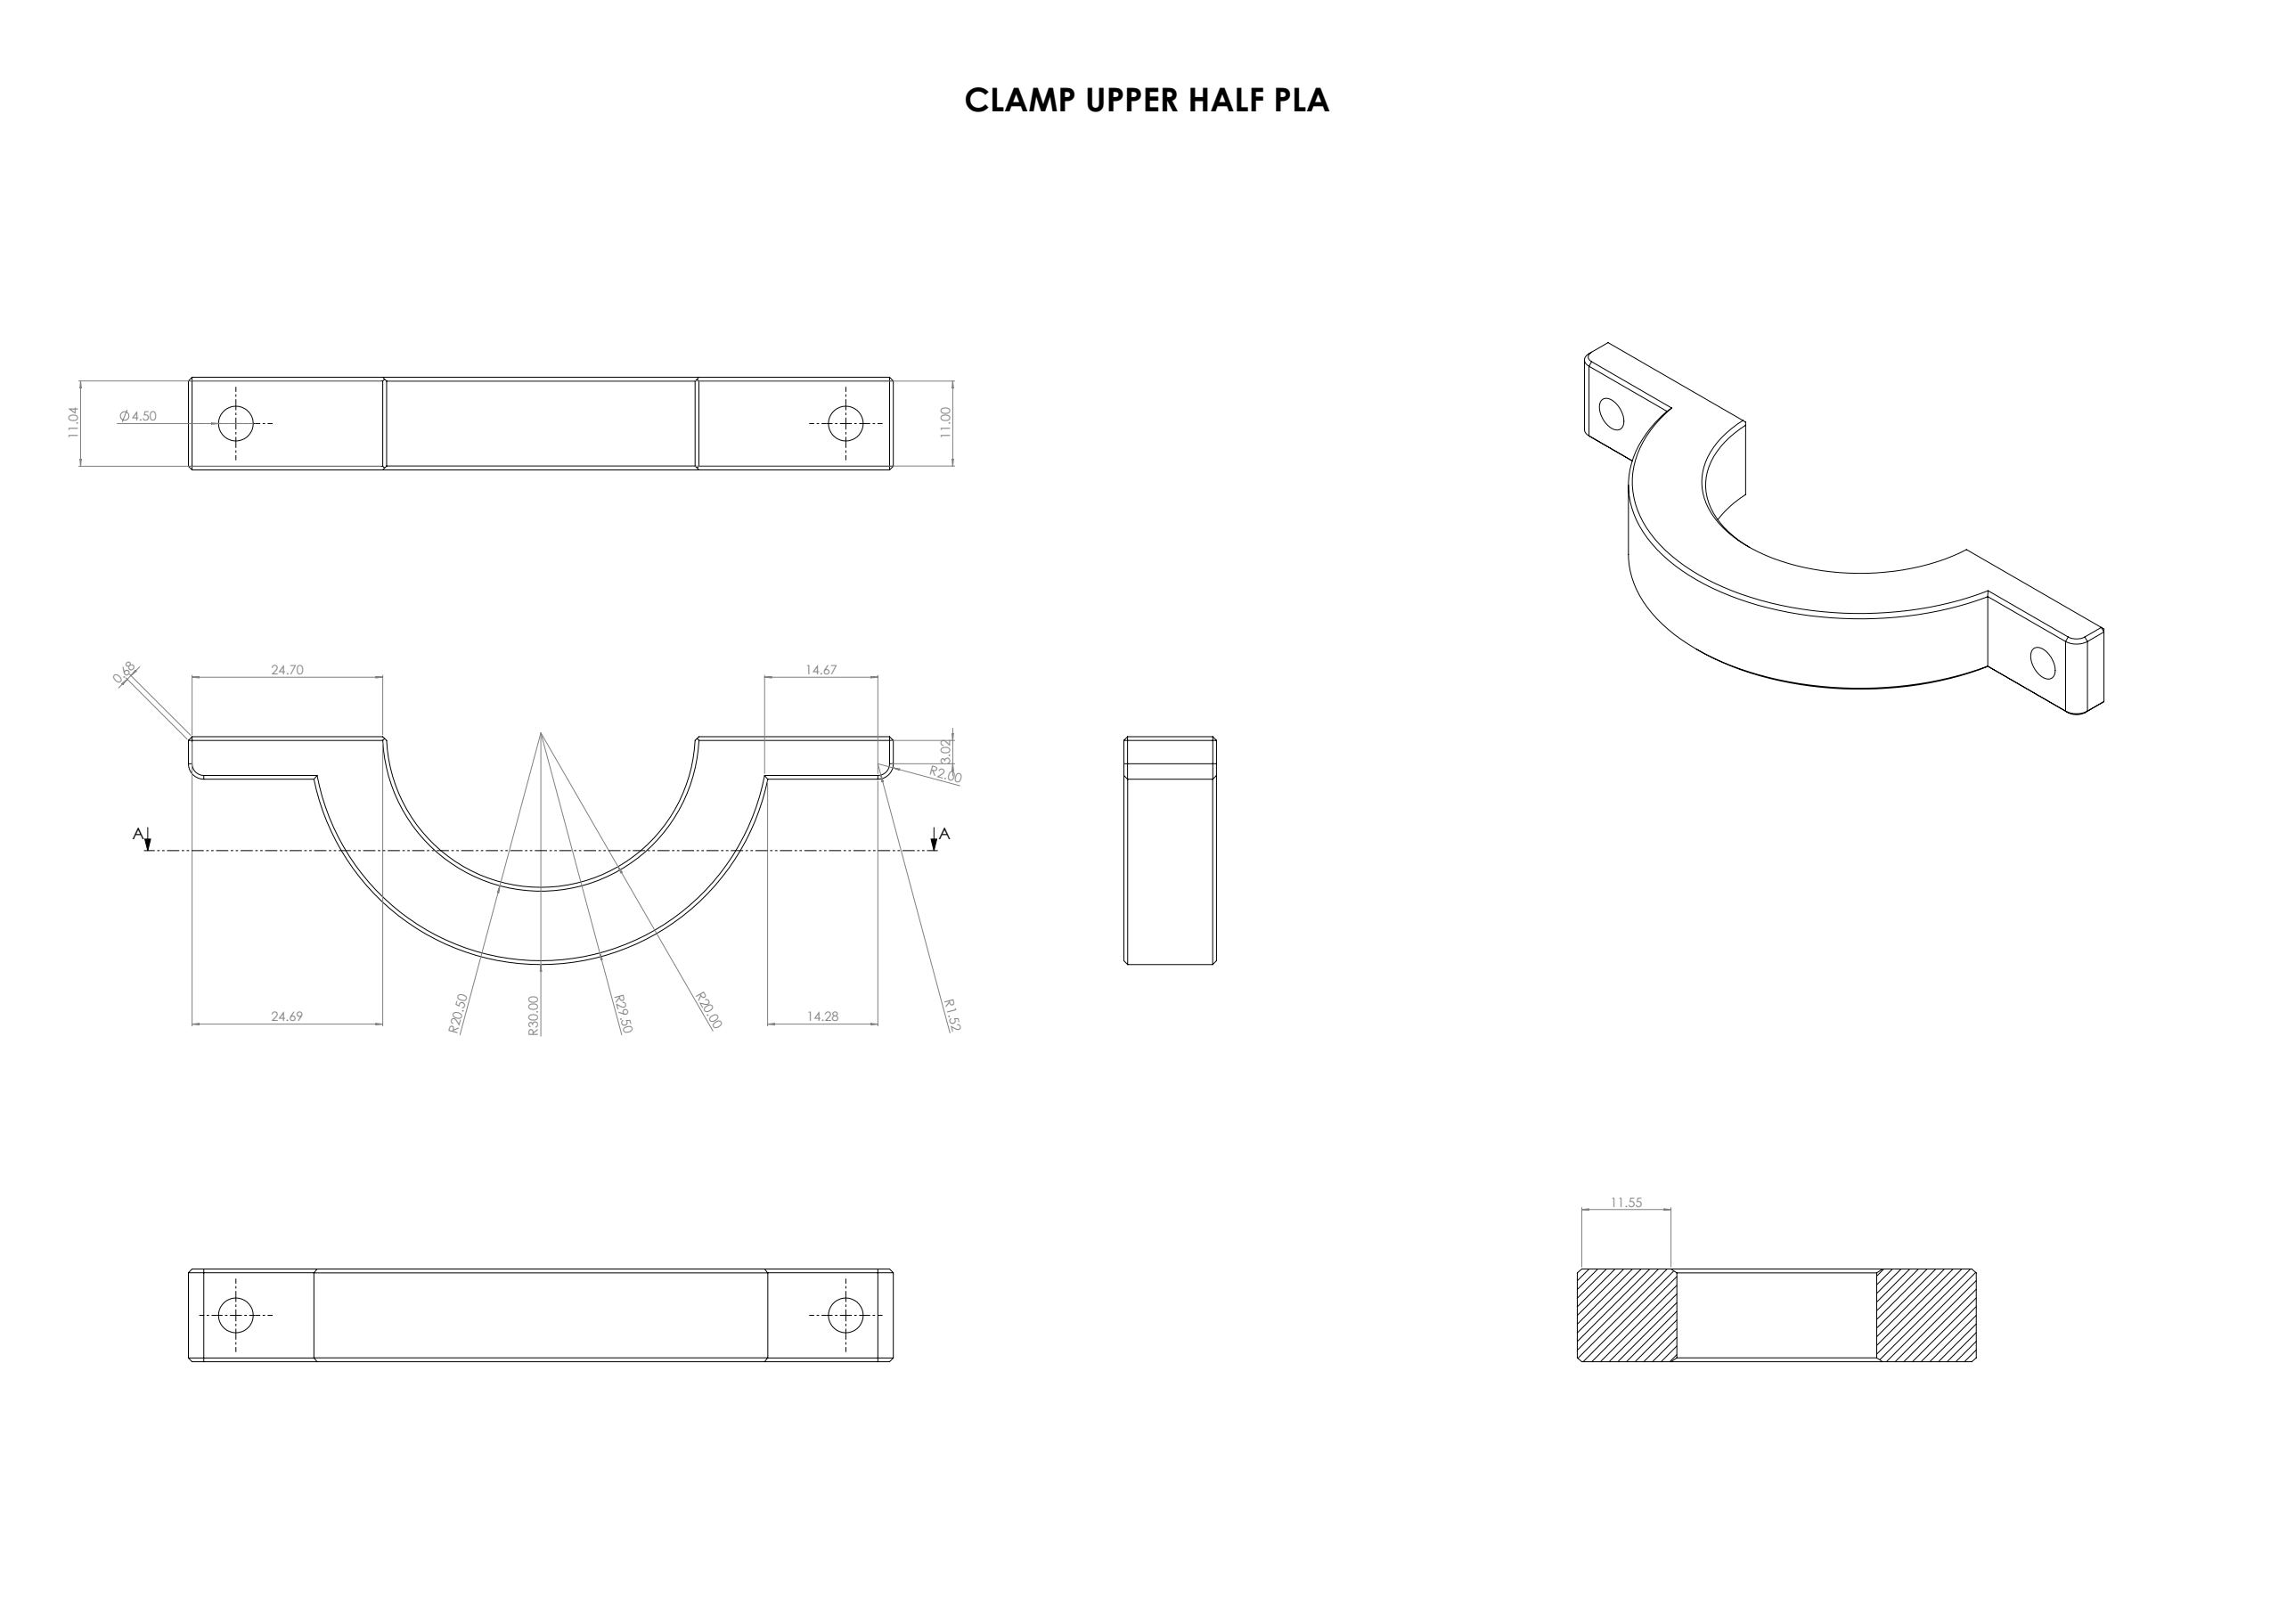
ISO-10303-21;
HEADER;
/* Generated by software containing ST-Developer
 * from STEP Tools, Inc. (www.steptools.com) 
 */

FILE_DESCRIPTION(
/* description */ (''),
/* implementation_level */ '2;1');

FILE_NAME(
/* name */ '01_Clamp_Upper_Half_PLA.step',
/* time_stamp */ '2026-10-21T02:01:14-07:00',
/* author */ (''),
/* organization */ (''),
/* preprocessor_version */ 'ST-DEVELOPER v20.2',
/* originating_system */ 'Autodesk Translation Framework v15.15.0.0',
/* authorisation */ '');

FILE_SCHEMA (('AUTOMOTIVE_DESIGN { 1 0 10303 214 3 1 1 }'));
ENDSEC;

DATA;
#10=MECHANICAL_DESIGN_GEOMETRIC_PRESENTATION_REPRESENTATION('',(#614),#37181);
#588=SHAPE_REPRESENTATION_RELATIONSHIP('SRR','None',#37238,#601);
#601=ADVANCED_BREP_SHAPE_REPRESENTATION('',(#627),#37168);
#614=STYLED_ITEM('',(#37359),#627);
#627=MANIFOLD_SOLID_BREP('Body1',#14776);
#640=FACE_BOUND('',#2226,.T.);
#641=FACE_BOUND('',#2241,.T.);
#642=FACE_BOUND('',#2250,.T.);
#643=FACE_BOUND('',#2253,.T.);
#690=CYLINDRICAL_SURFACE('',#14940,20.);
#691=CYLINDRICAL_SURFACE('',#14961,2.);
#692=CYLINDRICAL_SURFACE('',#14987,30.);
#693=CYLINDRICAL_SURFACE('',#14988,2.25);
#694=CYLINDRICAL_SURFACE('',#14990,2.25);
#695=CYLINDRICAL_SURFACE('',#14993,2.);
#951=CIRCLE('',#14938,20.);
#952=CIRCLE('',#14939,20.5);
#953=CIRCLE('',#14941,20.);
#954=CIRCLE('',#14946,2.);
#955=CIRCLE('',#14947,1.52);
#956=CIRCLE('',#14953,2.);
#957=CIRCLE('',#14954,1.52);
#958=CIRCLE('',#14957,29.5);
#959=CIRCLE('',#14958,1.52);
#960=CIRCLE('',#14959,20.5);
#961=CIRCLE('',#14963,2.25);
#962=CIRCLE('',#14971,2.);
#963=CIRCLE('',#14976,2.);
#964=CIRCLE('',#14977,1.52);
#965=CIRCLE('',#14981,2.25);
#966=CIRCLE('',#14983,30.);
#967=CIRCLE('',#14985,30.);
#968=CIRCLE('',#14986,29.5);
#969=CIRCLE('',#14989,2.25);
#970=CIRCLE('',#14991,2.25);
#1283=CONICAL_SURFACE('',#14937,20.25,0.785398163397446);
#1284=CONICAL_SURFACE('',#14945,1.76,0.78539816339745);
#1285=CONICAL_SURFACE('',#14952,1.76,0.78539816339745);
#1286=CONICAL_SURFACE('',#14970,1.76,0.785398163397452);
#1287=CONICAL_SURFACE('',#14975,1.76,0.785398163397452);
#1288=CONICAL_SURFACE('',#14979,20.25,0.785398163397446);
#1289=CONICAL_SURFACE('',#14982,29.75,0.785398163397446);
#1290=CONICAL_SURFACE('',#14984,29.75,0.785398163397446);
#1368=FACE_OUTER_BOUND('',#2208,.T.);
#1369=FACE_OUTER_BOUND('',#2209,.T.);
#1370=FACE_OUTER_BOUND('',#2210,.T.);
#1371=FACE_OUTER_BOUND('',#2211,.T.);
#1372=FACE_OUTER_BOUND('',#2212,.T.);
#1373=FACE_OUTER_BOUND('',#2213,.T.);
#1374=FACE_OUTER_BOUND('',#2214,.T.);
#1375=FACE_OUTER_BOUND('',#2215,.T.);
#1376=FACE_OUTER_BOUND('',#2216,.T.);
#1377=FACE_OUTER_BOUND('',#2217,.T.);
#1378=FACE_OUTER_BOUND('',#2218,.T.);
#1379=FACE_OUTER_BOUND('',#2219,.T.);
#1380=FACE_OUTER_BOUND('',#2220,.T.);
#1381=FACE_OUTER_BOUND('',#2221,.T.);
#1382=FACE_OUTER_BOUND('',#2222,.T.);
#1383=FACE_OUTER_BOUND('',#2223,.T.);
#1384=FACE_OUTER_BOUND('',#2224,.T.);
#1385=FACE_OUTER_BOUND('',#2225,.T.);
#1386=FACE_OUTER_BOUND('',#2227,.T.);
#1387=FACE_OUTER_BOUND('',#2228,.T.);
#1388=FACE_OUTER_BOUND('',#2229,.T.);
#1389=FACE_OUTER_BOUND('',#2230,.T.);
#1390=FACE_OUTER_BOUND('',#2231,.T.);
#1391=FACE_OUTER_BOUND('',#2232,.T.);
#1392=FACE_OUTER_BOUND('',#2233,.T.);
#1393=FACE_OUTER_BOUND('',#2234,.T.);
#1394=FACE_OUTER_BOUND('',#2235,.T.);
#1395=FACE_OUTER_BOUND('',#2236,.T.);
#1396=FACE_OUTER_BOUND('',#2237,.T.);
#1397=FACE_OUTER_BOUND('',#2238,.T.);
#1398=FACE_OUTER_BOUND('',#2239,.T.);
#1399=FACE_OUTER_BOUND('',#2240,.T.);
#1400=FACE_OUTER_BOUND('',#2242,.T.);
#1401=FACE_OUTER_BOUND('',#2243,.T.);
#1402=FACE_OUTER_BOUND('',#2244,.T.);
#1403=FACE_OUTER_BOUND('',#2245,.T.);
#1404=FACE_OUTER_BOUND('',#2246,.T.);
#1405=FACE_OUTER_BOUND('',#2247,.T.);
#1406=FACE_OUTER_BOUND('',#2248,.T.);
#1407=FACE_OUTER_BOUND('',#2249,.T.);
#1408=FACE_OUTER_BOUND('',#2251,.T.);
#1409=FACE_OUTER_BOUND('',#2252,.T.);
#2208=EDGE_LOOP('',(#9171,#9172,#9173,#9174,#9175,#9176));
#2209=EDGE_LOOP('',(#9177,#9178,#9179,#9180,#9181));
#2210=EDGE_LOOP('',(#9182,#9183,#9184,#9185,#9186,#9187));
#2211=EDGE_LOOP('',(#9188,#9189,#9190,#9191));
#2212=EDGE_LOOP('',(#9192,#9193,#9194));
#2213=EDGE_LOOP('',(#9195,#9196,#9197));
#2214=EDGE_LOOP('',(#9198,#9199,#9200,#9201));
#2215=EDGE_LOOP('',(#9202,#9203,#9204,#9205));
#2216=EDGE_LOOP('',(#9206,#9207,#9208,#9209));
#2217=EDGE_LOOP('',(#9210,#9211,#9212,#9213,#9214));
#2218=EDGE_LOOP('',(#9215,#9216,#9217,#9218));
#2219=EDGE_LOOP('',(#9219,#9220,#9221,#9222));
#2220=EDGE_LOOP('',(#9223,#9224,#9225,#9226));
#2221=EDGE_LOOP('',(#9227,#9228,#9229,#9230));
#2222=EDGE_LOOP('',(#9231,#9232,#9233,#9234,#9235,#9236,#9237,#9238,#9239,
#9240));
#2223=EDGE_LOOP('',(#9241,#9242,#9243,#9244));
#2224=EDGE_LOOP('',(#9245,#9246,#9247,#9248));
#2225=EDGE_LOOP('',(#9249,#9250,#9251,#9252,#9253,#9254));
#2226=EDGE_LOOP('',(#9255));
#2227=EDGE_LOOP('',(#9256,#9257,#9258,#9259,#9260,#9261));
#2228=EDGE_LOOP('',(#9262,#9263,#9264,#9265,#9266));
#2229=EDGE_LOOP('',(#9267,#9268,#9269));
#2230=EDGE_LOOP('',(#9270,#9271,#9272));
#2231=EDGE_LOOP('',(#9273,#9274,#9275,#9276,#9277));
#2232=EDGE_LOOP('',(#9278,#9279,#9280,#9281));
#2233=EDGE_LOOP('',(#9282,#9283,#9284,#9285));
#2234=EDGE_LOOP('',(#9286,#9287,#9288,#9289));
#2235=EDGE_LOOP('',(#9290,#9291,#9292,#9293));
#2236=EDGE_LOOP('',(#9294,#9295,#9296,#9297));
#2237=EDGE_LOOP('',(#9298,#9299,#9300,#9301));
#2238=EDGE_LOOP('',(#9302,#9303,#9304,#9305));
#2239=EDGE_LOOP('',(#9306,#9307,#9308,#9309,#9310,#9311));
#2240=EDGE_LOOP('',(#9312,#9313,#9314,#9315));
#2241=EDGE_LOOP('',(#9316));
#2242=EDGE_LOOP('',(#9317,#9318,#9319,#9320,#9321,#9322));
#2243=EDGE_LOOP('',(#9323,#9324,#9325,#9326,#9327,#9328));
#2244=EDGE_LOOP('',(#9329,#9330,#9331,#9332));
#2245=EDGE_LOOP('',(#9333,#9334,#9335,#9336));
#2246=EDGE_LOOP('',(#9337,#9338,#9339,#9340));
#2247=EDGE_LOOP('',(#9341,#9342,#9343,#9344,#9345,#9346,#9347,#9348,#9349,
#9350));
#2248=EDGE_LOOP('',(#9351,#9352,#9353,#9354));
#2249=EDGE_LOOP('',(#9355,#9356,#9357,#9358,#9359,#9360));
#2250=EDGE_LOOP('',(#9361));
#2251=EDGE_LOOP('',(#9362,#9363,#9364,#9365));
#2252=EDGE_LOOP('',(#9366,#9367,#9368,#9369));
#2253=EDGE_LOOP('',(#9370));
#3098=(
BOUNDED_CURVE()
B_SPLINE_CURVE(2,(#19759,#19760,#19761),.UNSPECIFIED.,.F.,.F.)
B_SPLINE_CURVE_WITH_KNOTS((3,3),(0.0434191036447886,0.0876516150043351),
 .UNSPECIFIED.)
CURVE()
GEOMETRIC_REPRESENTATION_ITEM()
RATIONAL_B_SPLINE_CURVE((1.00007900493244,1.00007974496639,1.))
REPRESENTATION_ITEM('')
);
#3099=(
BOUNDED_CURVE()
B_SPLINE_CURVE(2,(#19764,#19765,#19766),.UNSPECIFIED.,.F.,.F.)
B_SPLINE_CURVE_WITH_KNOTS((3,3),(0.,0.0442325113595662),.UNSPECIFIED.)
CURVE()
GEOMETRIC_REPRESENTATION_ITEM()
RATIONAL_B_SPLINE_CURVE((1.,1.00007974496581,1.00007900493187))
REPRESENTATION_ITEM('')
);
#3100=(
BOUNDED_CURVE()
B_SPLINE_CURVE(2,(#19769,#19770,#19771),.UNSPECIFIED.,.F.,.F.)
B_SPLINE_CURVE_WITH_KNOTS((3,3),(0.0429017134859095,0.085594459730905),
 .UNSPECIFIED.)
CURVE()
GEOMETRIC_REPRESENTATION_ITEM()
RATIONAL_B_SPLINE_CURVE((1.,1.,1.))
REPRESENTATION_ITEM('')
);
#3101=(
BOUNDED_CURVE()
B_SPLINE_CURVE(2,(#19781,#19782,#19783),.UNSPECIFIED.,.F.,.F.)
B_SPLINE_CURVE_WITH_KNOTS((3,3),(0.0434191036447867,0.0876516150043353),
 .UNSPECIFIED.)
CURVE()
GEOMETRIC_REPRESENTATION_ITEM()
RATIONAL_B_SPLINE_CURVE((1.00007900493282,1.00007974496678,1.))
REPRESENTATION_ITEM('')
);
#3102=(
BOUNDED_CURVE()
B_SPLINE_CURVE(2,(#19785,#19786,#19787),.UNSPECIFIED.,.F.,.F.)
B_SPLINE_CURVE_WITH_KNOTS((3,3),(0.,0.0426927462450535),.UNSPECIFIED.)
CURVE()
GEOMETRIC_REPRESENTATION_ITEM()
RATIONAL_B_SPLINE_CURVE((1.,1.,1.))
REPRESENTATION_ITEM('')
);
#3103=(
BOUNDED_CURVE()
B_SPLINE_CURVE(2,(#19819,#19820,#19821),.UNSPECIFIED.,.F.,.F.)
B_SPLINE_CURVE_WITH_KNOTS((3,3),(0.,0.0785138217700896),.UNSPECIFIED.)
CURVE()
GEOMETRIC_REPRESENTATION_ITEM()
RATIONAL_B_SPLINE_CURVE((1.,1.,1.))
REPRESENTATION_ITEM('')
);
#3104=(
BOUNDED_CURVE()
B_SPLINE_CURVE(2,(#19828,#19829,#19830),.UNSPECIFIED.,.F.,.F.)
B_SPLINE_CURVE_WITH_KNOTS((3,3),(0.,0.0426927462450536),.UNSPECIFIED.)
CURVE()
GEOMETRIC_REPRESENTATION_ITEM()
RATIONAL_B_SPLINE_CURVE((1.,1.,1.))
REPRESENTATION_ITEM('')
);
#3105=(
BOUNDED_CURVE()
B_SPLINE_CURVE(2,(#19837,#19838,#19839),.UNSPECIFIED.,.F.,.F.)
B_SPLINE_CURVE_WITH_KNOTS((3,3),(0.,0.0785138217700896),.UNSPECIFIED.)
CURVE()
GEOMETRIC_REPRESENTATION_ITEM()
RATIONAL_B_SPLINE_CURVE((1.,1.,1.))
REPRESENTATION_ITEM('')
);
#3106=(
BOUNDED_CURVE()
B_SPLINE_CURVE(2,(#19872,#19873,#19874),.UNSPECIFIED.,.F.,.F.)
B_SPLINE_CURVE_WITH_KNOTS((3,3),(0.0686220150831262,0.071456332389423),
 .UNSPECIFIED.)
CURVE()
GEOMETRIC_REPRESENTATION_ITEM()
RATIONAL_B_SPLINE_CURVE((1.00000280409598,1.00000145995723,1.))
REPRESENTATION_ITEM('')
);
#3107=(
BOUNDED_CURVE()
B_SPLINE_CURVE(2,(#19877,#19878,#19879),.UNSPECIFIED.,.F.,.F.)
B_SPLINE_CURVE_WITH_KNOTS((3,3),(0.,0.00283431730629652),.UNSPECIFIED.)
CURVE()
GEOMETRIC_REPRESENTATION_ITEM()
RATIONAL_B_SPLINE_CURVE((1.,1.00000145995723,1.00000280409598))
REPRESENTATION_ITEM('')
);
#3108=(
BOUNDED_CURVE()
B_SPLINE_CURVE(2,(#19889,#19890,#19891),.UNSPECIFIED.,.F.,.F.)
B_SPLINE_CURVE_WITH_KNOTS((3,3),(0.,0.0442325113595461),.UNSPECIFIED.)
CURVE()
GEOMETRIC_REPRESENTATION_ITEM()
RATIONAL_B_SPLINE_CURVE((1.,1.00007974496639,1.00007900493244))
REPRESENTATION_ITEM('')
);
#3109=(
BOUNDED_CURVE()
B_SPLINE_CURVE(2,(#19909,#19910,#19911),.UNSPECIFIED.,.F.,.F.)
B_SPLINE_CURVE_WITH_KNOTS((3,3),(0.0429017134859048,0.0855944597309048),
 .UNSPECIFIED.)
CURVE()
GEOMETRIC_REPRESENTATION_ITEM()
RATIONAL_B_SPLINE_CURVE((1.,1.,1.))
REPRESENTATION_ITEM('')
);
#3110=(
BOUNDED_CURVE()
B_SPLINE_CURVE(2,(#19915,#19916,#19917),.UNSPECIFIED.,.F.,.F.)
B_SPLINE_CURVE_WITH_KNOTS((3,3),(0.,0.0785138217700896),.UNSPECIFIED.)
CURVE()
GEOMETRIC_REPRESENTATION_ITEM()
RATIONAL_B_SPLINE_CURVE((1.,1.,1.))
REPRESENTATION_ITEM('')
);
#3111=(
BOUNDED_CURVE()
B_SPLINE_CURVE(2,(#19945,#19946,#19947),.UNSPECIFIED.,.F.,.F.)
B_SPLINE_CURVE_WITH_KNOTS((3,3),(0.,0.0785138217700896),.UNSPECIFIED.)
CURVE()
GEOMETRIC_REPRESENTATION_ITEM()
RATIONAL_B_SPLINE_CURVE((1.,1.,1.))
REPRESENTATION_ITEM('')
);
#3112=(
BOUNDED_CURVE()
B_SPLINE_CURVE(2,(#19956,#19957,#19958),.UNSPECIFIED.,.F.,.F.)
B_SPLINE_CURVE_WITH_KNOTS((3,3),(0.0686220150831262,0.071456332389423),
 .UNSPECIFIED.)
CURVE()
GEOMETRIC_REPRESENTATION_ITEM()
RATIONAL_B_SPLINE_CURVE((1.00000280409598,1.00000145995723,1.))
REPRESENTATION_ITEM('')
);
#3113=(
BOUNDED_CURVE()
B_SPLINE_CURVE(2,(#19962,#19963,#19964),.UNSPECIFIED.,.F.,.F.)
B_SPLINE_CURVE_WITH_KNOTS((3,3),(0.,0.00283431730629652),.UNSPECIFIED.)
CURVE()
GEOMETRIC_REPRESENTATION_ITEM()
RATIONAL_B_SPLINE_CURVE((1.,1.00000145995723,1.00000280409598))
REPRESENTATION_ITEM('')
);
#3203=LINE('',#19753,#4442);
#3204=LINE('',#19755,#4443);
#3205=LINE('',#19757,#4444);
#3206=LINE('',#19763,#4445);
#3207=LINE('',#19773,#4446);
#3208=LINE('',#19775,#4447);
#3209=LINE('',#19776,#4448);
#3210=LINE('',#19792,#4449);
#3211=LINE('',#19795,#4450);
#3212=LINE('',#19796,#4451);
#3213=LINE('',#19800,#4452);
#3214=LINE('',#19802,#4453);
#3215=LINE('',#19803,#4454);
#3216=LINE('',#19807,#4455);
#3217=LINE('',#19808,#4456);
#3218=LINE('',#19809,#4457);
#3219=LINE('',#19814,#4458);
#3220=LINE('',#19822,#4459);
#3221=LINE('',#19823,#4460);
#3222=LINE('',#19825,#4461);
#3223=LINE('',#19827,#4462);
#3224=LINE('',#19832,#4463);
#3225=LINE('',#19833,#4464);
#3226=LINE('',#19841,#4465);
#3227=LINE('',#19843,#4466);
#3228=LINE('',#19844,#4467);
#3229=LINE('',#19849,#4468);
#3230=LINE('',#19852,#4469);
#3231=LINE('',#19853,#4470);
#3232=LINE('',#19858,#4471);
#3233=LINE('',#19862,#4472);
#3234=LINE('',#19864,#4473);
#3235=LINE('',#19867,#4474);
#3236=LINE('',#19869,#4475);
#3237=LINE('',#19876,#4476);
#3238=LINE('',#19885,#4477);
#3239=LINE('',#19887,#4478);
#3240=LINE('',#19888,#4479);
#3241=LINE('',#19894,#4480);
#3242=LINE('',#19896,#4481);
#3243=LINE('',#19897,#4482);
#3244=LINE('',#19900,#4483);
#3245=LINE('',#19901,#4484);
#3246=LINE('',#19905,#4485);
#3247=LINE('',#19906,#4486);
#3248=LINE('',#19907,#4487);
#3249=LINE('',#19912,#4488);
#3250=LINE('',#19919,#4489);
#3251=LINE('',#19920,#4490);
#3252=LINE('',#19924,#4491);
#3253=LINE('',#19926,#4492);
#3254=LINE('',#19928,#4493);
#3255=LINE('',#19929,#4494);
#3256=LINE('',#19933,#4495);
#3257=LINE('',#19934,#4496);
#3258=LINE('',#19935,#4497);
#3259=LINE('',#19940,#4498);
#3260=LINE('',#19948,#4499);
#3261=LINE('',#19949,#4500);
#3262=LINE('',#19968,#4501);
#3263=LINE('',#19971,#4502);
#3264=LINE('',#19976,#4503);
#3265=LINE('',#19979,#4504);
#3266=LINE('',#19980,#4505);
#4442=VECTOR('',#16131,10.);
#4443=VECTOR('',#16132,10.);
#4444=VECTOR('',#16133,10.);
#4445=VECTOR('',#16134,10.);
#4446=VECTOR('',#16137,10.);
#4447=VECTOR('',#16138,10.);
#4448=VECTOR('',#16139,10.);
#4449=VECTOR('',#16150,10.);
#4450=VECTOR('',#16153,10.);
#4451=VECTOR('',#16154,10.);
#4452=VECTOR('',#16157,10.);
#4453=VECTOR('',#16158,10.);
#4454=VECTOR('',#16159,10.);
#4455=VECTOR('',#16162,10.);
#4456=VECTOR('',#16163,10.);
#4457=VECTOR('',#16164,10.);
#4458=VECTOR('',#16169,10.);
#4459=VECTOR('',#16174,10.);
#4460=VECTOR('',#16175,10.);
#4461=VECTOR('',#16178,10.);
#4462=VECTOR('',#16179,10.);
#4463=VECTOR('',#16182,10.);
#4464=VECTOR('',#16183,10.);
#4465=VECTOR('',#16186,10.);
#4466=VECTOR('',#16187,10.);
#4467=VECTOR('',#16188,10.);
#4468=VECTOR('',#16193,10.);
#4469=VECTOR('',#16198,10.);
#4470=VECTOR('',#16199,10.);
#4471=VECTOR('',#16204,10.);
#4472=VECTOR('',#16207,10.);
#4473=VECTOR('',#16208,10.);
#4474=VECTOR('',#16213,10.);
#4475=VECTOR('',#16216,10.);
#4476=VECTOR('',#16219,10.);
#4477=VECTOR('',#16224,10.);
#4478=VECTOR('',#16225,10.);
#4479=VECTOR('',#16226,10.);
#4480=VECTOR('',#16229,10.);
#4481=VECTOR('',#16230,10.);
#4482=VECTOR('',#16231,10.);
#4483=VECTOR('',#16234,10.);
#4484=VECTOR('',#16235,10.);
#4485=VECTOR('',#16238,10.);
#4486=VECTOR('',#16239,10.);
#4487=VECTOR('',#16240,10.);
#4488=VECTOR('',#16243,10.);
#4489=VECTOR('',#16246,10.);
#4490=VECTOR('',#16247,10.);
#4491=VECTOR('',#16252,10.);
#4492=VECTOR('',#16255,10.);
#4493=VECTOR('',#16258,10.);
#4494=VECTOR('',#16259,10.);
#4495=VECTOR('',#16262,10.);
#4496=VECTOR('',#16263,10.);
#4497=VECTOR('',#16264,10.);
#4498=VECTOR('',#16269,10.);
#4499=VECTOR('',#16274,10.);
#4500=VECTOR('',#16275,10.);
#4501=VECTOR('',#16294,10.);
#4502=VECTOR('',#16297,2.25);
#4503=VECTOR('',#16304,2.25);
#4504=VECTOR('',#16309,10.);
#4505=VECTOR('',#16310,10.);
#5681=VERTEX_POINT('',#19751);
#5682=VERTEX_POINT('',#19752);
#5683=VERTEX_POINT('',#19754);
#5684=VERTEX_POINT('',#19756);
#5685=VERTEX_POINT('',#19758);
#5686=VERTEX_POINT('',#19762);
#5687=VERTEX_POINT('',#19768);
#5688=VERTEX_POINT('',#19772);
#5689=VERTEX_POINT('',#19774);
#5690=VERTEX_POINT('',#19778);
#5691=VERTEX_POINT('',#19780);
#5692=VERTEX_POINT('',#19784);
#5693=VERTEX_POINT('',#19790);
#5694=VERTEX_POINT('',#19794);
#5695=VERTEX_POINT('',#19798);
#5696=VERTEX_POINT('',#19799);
#5697=VERTEX_POINT('',#19801);
#5698=VERTEX_POINT('',#19805);
#5699=VERTEX_POINT('',#19806);
#5700=VERTEX_POINT('',#19811);
#5701=VERTEX_POINT('',#19813);
#5702=VERTEX_POINT('',#19817);
#5703=VERTEX_POINT('',#19818);
#5704=VERTEX_POINT('',#19826);
#5705=VERTEX_POINT('',#19835);
#5706=VERTEX_POINT('',#19836);
#5707=VERTEX_POINT('',#19840);
#5708=VERTEX_POINT('',#19842);
#5709=VERTEX_POINT('',#19846);
#5710=VERTEX_POINT('',#19848);
#5711=VERTEX_POINT('',#19855);
#5712=VERTEX_POINT('',#19857);
#5713=VERTEX_POINT('',#19859);
#5714=VERTEX_POINT('',#19861);
#5715=VERTEX_POINT('',#19863);
#5716=VERTEX_POINT('',#19871);
#5717=VERTEX_POINT('',#19875);
#5718=VERTEX_POINT('',#19880);
#5719=VERTEX_POINT('',#19883);
#5720=VERTEX_POINT('',#19884);
#5721=VERTEX_POINT('',#19886);
#5722=VERTEX_POINT('',#19893);
#5723=VERTEX_POINT('',#19895);
#5724=VERTEX_POINT('',#19899);
#5725=VERTEX_POINT('',#19903);
#5726=VERTEX_POINT('',#19904);
#5727=VERTEX_POINT('',#19914);
#5728=VERTEX_POINT('',#19918);
#5729=VERTEX_POINT('',#19922);
#5730=VERTEX_POINT('',#19931);
#5731=VERTEX_POINT('',#19932);
#5732=VERTEX_POINT('',#19937);
#5733=VERTEX_POINT('',#19939);
#5734=VERTEX_POINT('',#19943);
#5735=VERTEX_POINT('',#19944);
#5736=VERTEX_POINT('',#19952);
#5737=VERTEX_POINT('',#19955);
#5738=VERTEX_POINT('',#19961);
#5739=VERTEX_POINT('',#19970);
#5740=VERTEX_POINT('',#19974);
#7027=EDGE_CURVE('',#5681,#5682,#3203,.T.);
#7028=EDGE_CURVE('',#5682,#5683,#3204,.T.);
#7029=EDGE_CURVE('',#5683,#5684,#3205,.T.);
#7030=EDGE_CURVE('',#5684,#5685,#3098,.T.);
#7031=EDGE_CURVE('',#5685,#5686,#3206,.T.);
#7032=EDGE_CURVE('',#5686,#5681,#3099,.T.);
#7033=EDGE_CURVE('',#5681,#5687,#3100,.T.);
#7034=EDGE_CURVE('',#5687,#5688,#3207,.T.);
#7035=EDGE_CURVE('',#5688,#5689,#3208,.T.);
#7036=EDGE_CURVE('',#5689,#5682,#3209,.T.);
#7037=EDGE_CURVE('',#5686,#5690,#951,.T.);
#7038=EDGE_CURVE('',#5691,#5690,#3101,.T.);
#7039=EDGE_CURVE('',#5692,#5691,#3102,.T.);
#7040=EDGE_CURVE('',#5692,#5687,#952,.T.);
#7041=EDGE_CURVE('',#5693,#5685,#953,.T.);
#7042=EDGE_CURVE('',#5690,#5693,#3210,.T.);
#7043=EDGE_CURVE('',#5694,#5688,#3211,.T.);
#7044=EDGE_CURVE('',#5689,#5694,#3212,.T.);
#7045=EDGE_CURVE('',#5695,#5696,#3213,.T.);
#7046=EDGE_CURVE('',#5697,#5695,#3214,.T.);
#7047=EDGE_CURVE('',#5696,#5697,#3215,.T.);
#7048=EDGE_CURVE('',#5698,#5699,#3216,.T.);
#7049=EDGE_CURVE('',#5699,#5697,#3217,.T.);
#7050=EDGE_CURVE('',#5695,#5698,#3218,.T.);
#7051=EDGE_CURVE('',#5698,#5700,#954,.T.);
#7052=EDGE_CURVE('',#5700,#5701,#3219,.T.);
#7053=EDGE_CURVE('',#5701,#5699,#955,.T.);
#7054=EDGE_CURVE('',#5702,#5703,#3103,.F.);
#7055=EDGE_CURVE('',#5703,#5701,#3220,.T.);
#7056=EDGE_CURVE('',#5700,#5702,#3221,.T.);
#7057=EDGE_CURVE('',#5683,#5696,#3222,.T.);
#7058=EDGE_CURVE('',#5697,#5704,#3223,.T.);
#7059=EDGE_CURVE('',#5704,#5684,#3104,.T.);
#7060=EDGE_CURVE('',#5694,#5695,#3224,.T.);
#7061=EDGE_CURVE('',#5696,#5689,#3225,.T.);
#7062=EDGE_CURVE('',#5705,#5706,#3105,.F.);
#7063=EDGE_CURVE('',#5706,#5707,#3226,.T.);
#7064=EDGE_CURVE('',#5707,#5708,#3227,.T.);
#7065=EDGE_CURVE('',#5708,#5705,#3228,.T.);
#7066=EDGE_CURVE('',#5707,#5709,#956,.T.);
#7067=EDGE_CURVE('',#5709,#5710,#3229,.T.);
#7068=EDGE_CURVE('',#5710,#5708,#957,.T.);
#7069=EDGE_CURVE('',#5709,#5694,#3230,.T.);
#7070=EDGE_CURVE('',#5688,#5710,#3231,.T.);
#7071=EDGE_CURVE('',#5711,#5703,#958,.T.);
#7072=EDGE_CURVE('',#5712,#5711,#3232,.T.);
#7073=EDGE_CURVE('',#5713,#5712,#959,.T.);
#7074=EDGE_CURVE('',#5714,#5713,#3233,.T.);
#7075=EDGE_CURVE('',#5715,#5714,#3234,.T.);
#7076=EDGE_CURVE('',#5704,#5715,#960,.T.);
#7077=EDGE_CURVE('',#5698,#5709,#3235,.T.);
#7078=EDGE_CURVE('',#5707,#5700,#3236,.T.);
#7079=EDGE_CURVE('',#5716,#5706,#3106,.F.);
#7080=EDGE_CURVE('',#5717,#5716,#3237,.T.);
#7081=EDGE_CURVE('',#5702,#5717,#3107,.F.);
#7082=EDGE_CURVE('',#5718,#5718,#961,.T.);
#7083=EDGE_CURVE('',#5719,#5720,#3238,.T.);
#7084=EDGE_CURVE('',#5720,#5721,#3239,.T.);
#7085=EDGE_CURVE('',#5721,#5691,#3240,.T.);
#7086=EDGE_CURVE('',#5693,#5719,#3108,.T.);
#7087=EDGE_CURVE('',#5721,#5722,#3241,.T.);
#7088=EDGE_CURVE('',#5722,#5723,#3242,.T.);
#7089=EDGE_CURVE('',#5723,#5692,#3243,.T.);
#7090=EDGE_CURVE('',#5724,#5722,#3244,.T.);
#7091=EDGE_CURVE('',#5723,#5724,#3245,.T.);
#7092=EDGE_CURVE('',#5725,#5726,#3246,.T.);
#7093=EDGE_CURVE('',#5714,#5725,#3247,.T.);
#7094=EDGE_CURVE('',#5726,#5714,#3248,.T.);
#7095=EDGE_CURVE('',#5719,#5715,#3109,.T.);
#7096=EDGE_CURVE('',#5725,#5720,#3249,.T.);
#7097=EDGE_CURVE('',#5711,#5727,#3110,.F.);
#7098=EDGE_CURVE('',#5727,#5728,#3250,.T.);
#7099=EDGE_CURVE('',#5728,#5712,#3251,.T.);
#7100=EDGE_CURVE('',#5728,#5729,#962,.T.);
#7101=EDGE_CURVE('',#5729,#5713,#3252,.T.);
#7102=EDGE_CURVE('',#5729,#5726,#3253,.T.);
#7103=EDGE_CURVE('',#5722,#5725,#3254,.T.);
#7104=EDGE_CURVE('',#5726,#5724,#3255,.T.);
#7105=EDGE_CURVE('',#5730,#5731,#3256,.T.);
#7106=EDGE_CURVE('',#5731,#5723,#3257,.T.);
#7107=EDGE_CURVE('',#5724,#5730,#3258,.T.);
#7108=EDGE_CURVE('',#5730,#5732,#963,.T.);
#7109=EDGE_CURVE('',#5732,#5733,#3259,.T.);
#7110=EDGE_CURVE('',#5733,#5731,#964,.T.);
#7111=EDGE_CURVE('',#5734,#5735,#3111,.F.);
#7112=EDGE_CURVE('',#5735,#5733,#3260,.T.);
#7113=EDGE_CURVE('',#5732,#5734,#3261,.T.);
#7114=EDGE_CURVE('',#5736,#5736,#965,.T.);
#7115=EDGE_CURVE('',#5737,#5727,#3112,.F.);
#7116=EDGE_CURVE('',#5717,#5737,#966,.T.);
#7117=EDGE_CURVE('',#5734,#5738,#3113,.F.);
#7118=EDGE_CURVE('',#5738,#5716,#967,.T.);
#7119=EDGE_CURVE('',#5705,#5735,#968,.T.);
#7120=EDGE_CURVE('',#5737,#5738,#3262,.T.);
#7121=EDGE_CURVE('',#5718,#5739,#3263,.T.);
#7122=EDGE_CURVE('',#5739,#5739,#969,.T.);
#7123=EDGE_CURVE('',#5740,#5740,#970,.T.);
#7124=EDGE_CURVE('',#5740,#5736,#3264,.T.);
#7125=EDGE_CURVE('',#5728,#5732,#3265,.T.);
#7126=EDGE_CURVE('',#5730,#5729,#3266,.T.);
#9171=ORIENTED_EDGE('',*,*,#7027,.T.);
#9172=ORIENTED_EDGE('',*,*,#7028,.T.);
#9173=ORIENTED_EDGE('',*,*,#7029,.T.);
#9174=ORIENTED_EDGE('',*,*,#7030,.T.);
#9175=ORIENTED_EDGE('',*,*,#7031,.T.);
#9176=ORIENTED_EDGE('',*,*,#7032,.T.);
#9177=ORIENTED_EDGE('',*,*,#7027,.F.);
#9178=ORIENTED_EDGE('',*,*,#7033,.T.);
#9179=ORIENTED_EDGE('',*,*,#7034,.T.);
#9180=ORIENTED_EDGE('',*,*,#7035,.T.);
#9181=ORIENTED_EDGE('',*,*,#7036,.T.);
#9182=ORIENTED_EDGE('',*,*,#7032,.F.);
#9183=ORIENTED_EDGE('',*,*,#7037,.T.);
#9184=ORIENTED_EDGE('',*,*,#7038,.F.);
#9185=ORIENTED_EDGE('',*,*,#7039,.F.);
#9186=ORIENTED_EDGE('',*,*,#7040,.T.);
#9187=ORIENTED_EDGE('',*,*,#7033,.F.);
#9188=ORIENTED_EDGE('',*,*,#7031,.F.);
#9189=ORIENTED_EDGE('',*,*,#7041,.F.);
#9190=ORIENTED_EDGE('',*,*,#7042,.F.);
#9191=ORIENTED_EDGE('',*,*,#7037,.F.);
#9192=ORIENTED_EDGE('',*,*,#7043,.F.);
#9193=ORIENTED_EDGE('',*,*,#7044,.F.);
#9194=ORIENTED_EDGE('',*,*,#7035,.F.);
#9195=ORIENTED_EDGE('',*,*,#7045,.F.);
#9196=ORIENTED_EDGE('',*,*,#7046,.F.);
#9197=ORIENTED_EDGE('',*,*,#7047,.F.);
#9198=ORIENTED_EDGE('',*,*,#7048,.T.);
#9199=ORIENTED_EDGE('',*,*,#7049,.T.);
#9200=ORIENTED_EDGE('',*,*,#7046,.T.);
#9201=ORIENTED_EDGE('',*,*,#7050,.T.);
#9202=ORIENTED_EDGE('',*,*,#7048,.F.);
#9203=ORIENTED_EDGE('',*,*,#7051,.T.);
#9204=ORIENTED_EDGE('',*,*,#7052,.T.);
#9205=ORIENTED_EDGE('',*,*,#7053,.T.);
#9206=ORIENTED_EDGE('',*,*,#7054,.T.);
#9207=ORIENTED_EDGE('',*,*,#7055,.T.);
#9208=ORIENTED_EDGE('',*,*,#7052,.F.);
#9209=ORIENTED_EDGE('',*,*,#7056,.T.);
#9210=ORIENTED_EDGE('',*,*,#7029,.F.);
#9211=ORIENTED_EDGE('',*,*,#7057,.T.);
#9212=ORIENTED_EDGE('',*,*,#7047,.T.);
#9213=ORIENTED_EDGE('',*,*,#7058,.T.);
#9214=ORIENTED_EDGE('',*,*,#7059,.T.);
#9215=ORIENTED_EDGE('',*,*,#7044,.T.);
#9216=ORIENTED_EDGE('',*,*,#7060,.T.);
#9217=ORIENTED_EDGE('',*,*,#7045,.T.);
#9218=ORIENTED_EDGE('',*,*,#7061,.T.);
#9219=ORIENTED_EDGE('',*,*,#7062,.T.);
#9220=ORIENTED_EDGE('',*,*,#7063,.T.);
#9221=ORIENTED_EDGE('',*,*,#7064,.T.);
#9222=ORIENTED_EDGE('',*,*,#7065,.T.);
#9223=ORIENTED_EDGE('',*,*,#7064,.F.);
#9224=ORIENTED_EDGE('',*,*,#7066,.T.);
#9225=ORIENTED_EDGE('',*,*,#7067,.T.);
#9226=ORIENTED_EDGE('',*,*,#7068,.T.);
#9227=ORIENTED_EDGE('',*,*,#7067,.F.);
#9228=ORIENTED_EDGE('',*,*,#7069,.T.);
#9229=ORIENTED_EDGE('',*,*,#7043,.T.);
#9230=ORIENTED_EDGE('',*,*,#7070,.T.);
#9231=ORIENTED_EDGE('',*,*,#7058,.F.);
#9232=ORIENTED_EDGE('',*,*,#7049,.F.);
#9233=ORIENTED_EDGE('',*,*,#7053,.F.);
#9234=ORIENTED_EDGE('',*,*,#7055,.F.);
#9235=ORIENTED_EDGE('',*,*,#7071,.F.);
#9236=ORIENTED_EDGE('',*,*,#7072,.F.);
#9237=ORIENTED_EDGE('',*,*,#7073,.F.);
#9238=ORIENTED_EDGE('',*,*,#7074,.F.);
#9239=ORIENTED_EDGE('',*,*,#7075,.F.);
#9240=ORIENTED_EDGE('',*,*,#7076,.F.);
#9241=ORIENTED_EDGE('',*,*,#7050,.F.);
#9242=ORIENTED_EDGE('',*,*,#7060,.F.);
#9243=ORIENTED_EDGE('',*,*,#7069,.F.);
#9244=ORIENTED_EDGE('',*,*,#7077,.F.);
#9245=ORIENTED_EDGE('',*,*,#7051,.F.);
#9246=ORIENTED_EDGE('',*,*,#7077,.T.);
#9247=ORIENTED_EDGE('',*,*,#7066,.F.);
#9248=ORIENTED_EDGE('',*,*,#7078,.T.);
#9249=ORIENTED_EDGE('',*,*,#7056,.F.);
#9250=ORIENTED_EDGE('',*,*,#7078,.F.);
#9251=ORIENTED_EDGE('',*,*,#7063,.F.);
#9252=ORIENTED_EDGE('',*,*,#7079,.F.);
#9253=ORIENTED_EDGE('',*,*,#7080,.F.);
#9254=ORIENTED_EDGE('',*,*,#7081,.F.);
#9255=ORIENTED_EDGE('',*,*,#7082,.T.);
#9256=ORIENTED_EDGE('',*,*,#7083,.T.);
#9257=ORIENTED_EDGE('',*,*,#7084,.T.);
#9258=ORIENTED_EDGE('',*,*,#7085,.T.);
#9259=ORIENTED_EDGE('',*,*,#7038,.T.);
#9260=ORIENTED_EDGE('',*,*,#7042,.T.);
#9261=ORIENTED_EDGE('',*,*,#7086,.T.);
#9262=ORIENTED_EDGE('',*,*,#7085,.F.);
#9263=ORIENTED_EDGE('',*,*,#7087,.T.);
#9264=ORIENTED_EDGE('',*,*,#7088,.T.);
#9265=ORIENTED_EDGE('',*,*,#7089,.T.);
#9266=ORIENTED_EDGE('',*,*,#7039,.T.);
#9267=ORIENTED_EDGE('',*,*,#7088,.F.);
#9268=ORIENTED_EDGE('',*,*,#7090,.F.);
#9269=ORIENTED_EDGE('',*,*,#7091,.F.);
#9270=ORIENTED_EDGE('',*,*,#7092,.F.);
#9271=ORIENTED_EDGE('',*,*,#7093,.F.);
#9272=ORIENTED_EDGE('',*,*,#7094,.F.);
#9273=ORIENTED_EDGE('',*,*,#7083,.F.);
#9274=ORIENTED_EDGE('',*,*,#7095,.T.);
#9275=ORIENTED_EDGE('',*,*,#7075,.T.);
#9276=ORIENTED_EDGE('',*,*,#7093,.T.);
#9277=ORIENTED_EDGE('',*,*,#7096,.T.);
#9278=ORIENTED_EDGE('',*,*,#7097,.T.);
#9279=ORIENTED_EDGE('',*,*,#7098,.T.);
#9280=ORIENTED_EDGE('',*,*,#7099,.T.);
#9281=ORIENTED_EDGE('',*,*,#7072,.T.);
#9282=ORIENTED_EDGE('',*,*,#7099,.F.);
#9283=ORIENTED_EDGE('',*,*,#7100,.T.);
#9284=ORIENTED_EDGE('',*,*,#7101,.T.);
#9285=ORIENTED_EDGE('',*,*,#7073,.T.);
#9286=ORIENTED_EDGE('',*,*,#7101,.F.);
#9287=ORIENTED_EDGE('',*,*,#7102,.T.);
#9288=ORIENTED_EDGE('',*,*,#7094,.T.);
#9289=ORIENTED_EDGE('',*,*,#7074,.T.);
#9290=ORIENTED_EDGE('',*,*,#7090,.T.);
#9291=ORIENTED_EDGE('',*,*,#7103,.T.);
#9292=ORIENTED_EDGE('',*,*,#7092,.T.);
#9293=ORIENTED_EDGE('',*,*,#7104,.T.);
#9294=ORIENTED_EDGE('',*,*,#7105,.T.);
#9295=ORIENTED_EDGE('',*,*,#7106,.T.);
#9296=ORIENTED_EDGE('',*,*,#7091,.T.);
#9297=ORIENTED_EDGE('',*,*,#7107,.T.);
#9298=ORIENTED_EDGE('',*,*,#7105,.F.);
#9299=ORIENTED_EDGE('',*,*,#7108,.T.);
#9300=ORIENTED_EDGE('',*,*,#7109,.T.);
#9301=ORIENTED_EDGE('',*,*,#7110,.T.);
#9302=ORIENTED_EDGE('',*,*,#7111,.T.);
#9303=ORIENTED_EDGE('',*,*,#7112,.T.);
#9304=ORIENTED_EDGE('',*,*,#7109,.F.);
#9305=ORIENTED_EDGE('',*,*,#7113,.T.);
#9306=ORIENTED_EDGE('',*,*,#7030,.F.);
#9307=ORIENTED_EDGE('',*,*,#7059,.F.);
#9308=ORIENTED_EDGE('',*,*,#7076,.T.);
#9309=ORIENTED_EDGE('',*,*,#7095,.F.);
#9310=ORIENTED_EDGE('',*,*,#7086,.F.);
#9311=ORIENTED_EDGE('',*,*,#7041,.T.);
#9312=ORIENTED_EDGE('',*,*,#7084,.F.);
#9313=ORIENTED_EDGE('',*,*,#7096,.F.);
#9314=ORIENTED_EDGE('',*,*,#7103,.F.);
#9315=ORIENTED_EDGE('',*,*,#7087,.F.);
#9316=ORIENTED_EDGE('',*,*,#7114,.T.);
#9317=ORIENTED_EDGE('',*,*,#7115,.T.);
#9318=ORIENTED_EDGE('',*,*,#7097,.F.);
#9319=ORIENTED_EDGE('',*,*,#7071,.T.);
#9320=ORIENTED_EDGE('',*,*,#7054,.F.);
#9321=ORIENTED_EDGE('',*,*,#7081,.T.);
#9322=ORIENTED_EDGE('',*,*,#7116,.T.);
#9323=ORIENTED_EDGE('',*,*,#7117,.T.);
#9324=ORIENTED_EDGE('',*,*,#7118,.T.);
#9325=ORIENTED_EDGE('',*,*,#7079,.T.);
#9326=ORIENTED_EDGE('',*,*,#7062,.F.);
#9327=ORIENTED_EDGE('',*,*,#7119,.T.);
#9328=ORIENTED_EDGE('',*,*,#7111,.F.);
#9329=ORIENTED_EDGE('',*,*,#7116,.F.);
#9330=ORIENTED_EDGE('',*,*,#7080,.T.);
#9331=ORIENTED_EDGE('',*,*,#7118,.F.);
#9332=ORIENTED_EDGE('',*,*,#7120,.F.);
#9333=ORIENTED_EDGE('',*,*,#7082,.F.);
#9334=ORIENTED_EDGE('',*,*,#7121,.T.);
#9335=ORIENTED_EDGE('',*,*,#7122,.F.);
#9336=ORIENTED_EDGE('',*,*,#7121,.F.);
#9337=ORIENTED_EDGE('',*,*,#7123,.F.);
#9338=ORIENTED_EDGE('',*,*,#7124,.T.);
#9339=ORIENTED_EDGE('',*,*,#7114,.F.);
#9340=ORIENTED_EDGE('',*,*,#7124,.F.);
#9341=ORIENTED_EDGE('',*,*,#7034,.F.);
#9342=ORIENTED_EDGE('',*,*,#7040,.F.);
#9343=ORIENTED_EDGE('',*,*,#7089,.F.);
#9344=ORIENTED_EDGE('',*,*,#7106,.F.);
#9345=ORIENTED_EDGE('',*,*,#7110,.F.);
#9346=ORIENTED_EDGE('',*,*,#7112,.F.);
#9347=ORIENTED_EDGE('',*,*,#7119,.F.);
#9348=ORIENTED_EDGE('',*,*,#7065,.F.);
#9349=ORIENTED_EDGE('',*,*,#7068,.F.);
#9350=ORIENTED_EDGE('',*,*,#7070,.F.);
#9351=ORIENTED_EDGE('',*,*,#7100,.F.);
#9352=ORIENTED_EDGE('',*,*,#7125,.T.);
#9353=ORIENTED_EDGE('',*,*,#7108,.F.);
#9354=ORIENTED_EDGE('',*,*,#7126,.T.);
#9355=ORIENTED_EDGE('',*,*,#7098,.F.);
#9356=ORIENTED_EDGE('',*,*,#7115,.F.);
#9357=ORIENTED_EDGE('',*,*,#7120,.T.);
#9358=ORIENTED_EDGE('',*,*,#7117,.F.);
#9359=ORIENTED_EDGE('',*,*,#7113,.F.);
#9360=ORIENTED_EDGE('',*,*,#7125,.F.);
#9361=ORIENTED_EDGE('',*,*,#7123,.T.);
#9362=ORIENTED_EDGE('',*,*,#7102,.F.);
#9363=ORIENTED_EDGE('',*,*,#7126,.F.);
#9364=ORIENTED_EDGE('',*,*,#7107,.F.);
#9365=ORIENTED_EDGE('',*,*,#7104,.F.);
#9366=ORIENTED_EDGE('',*,*,#7028,.F.);
#9367=ORIENTED_EDGE('',*,*,#7036,.F.);
#9368=ORIENTED_EDGE('',*,*,#7061,.F.);
#9369=ORIENTED_EDGE('',*,*,#7057,.F.);
#9370=ORIENTED_EDGE('',*,*,#7122,.T.);
#13459=PLANE('',#14935);
#13460=PLANE('',#14936);
#13461=PLANE('',#14942);
#13462=PLANE('',#14943);
#13463=PLANE('',#14944);
#13464=PLANE('',#14948);
#13465=PLANE('',#14949);
#13466=PLANE('',#14950);
#13467=PLANE('',#14951);
#13468=PLANE('',#14955);
#13469=PLANE('',#14956);
#13470=PLANE('',#14960);
#13471=PLANE('',#14962);
#13472=PLANE('',#14964);
#13473=PLANE('',#14965);
#13474=PLANE('',#14966);
#13475=PLANE('',#14967);
#13476=PLANE('',#14968);
#13477=PLANE('',#14969);
#13478=PLANE('',#14972);
#13479=PLANE('',#14973);
#13480=PLANE('',#14974);
#13481=PLANE('',#14978);
#13482=PLANE('',#14980);
#13483=PLANE('',#14992);
#13484=PLANE('',#14994);
#13485=PLANE('',#14995);
#13486=PLANE('',#14996);
#13936=ADVANCED_FACE('',(#1368),#13459,.T.);
#13937=ADVANCED_FACE('',(#1369),#13460,.T.);
#13938=ADVANCED_FACE('',(#1370),#1283,.F.);
#13939=ADVANCED_FACE('',(#1371),#690,.F.);
#13940=ADVANCED_FACE('',(#1372),#13461,.T.);
#13941=ADVANCED_FACE('',(#1373),#13462,.T.);
#13942=ADVANCED_FACE('',(#1374),#13463,.T.);
#13943=ADVANCED_FACE('',(#1375),#1284,.T.);
#13944=ADVANCED_FACE('',(#1376),#13464,.T.);
#13945=ADVANCED_FACE('',(#1377),#13465,.T.);
#13946=ADVANCED_FACE('',(#1378),#13466,.T.);
#13947=ADVANCED_FACE('',(#1379),#13467,.T.);
#13948=ADVANCED_FACE('',(#1380),#1285,.T.);
#13949=ADVANCED_FACE('',(#1381),#13468,.T.);
#13950=ADVANCED_FACE('',(#1382),#13469,.F.);
#13951=ADVANCED_FACE('',(#1383),#13470,.T.);
#13952=ADVANCED_FACE('',(#1384),#691,.T.);
#13953=ADVANCED_FACE('',(#1385,#640),#13471,.T.);
#13954=ADVANCED_FACE('',(#1386),#13472,.T.);
#13955=ADVANCED_FACE('',(#1387),#13473,.T.);
#13956=ADVANCED_FACE('',(#1388),#13474,.T.);
#13957=ADVANCED_FACE('',(#1389),#13475,.T.);
#13958=ADVANCED_FACE('',(#1390),#13476,.T.);
#13959=ADVANCED_FACE('',(#1391),#13477,.T.);
#13960=ADVANCED_FACE('',(#1392),#1286,.T.);
#13961=ADVANCED_FACE('',(#1393),#13478,.T.);
#13962=ADVANCED_FACE('',(#1394),#13479,.T.);
#13963=ADVANCED_FACE('',(#1395),#13480,.T.);
#13964=ADVANCED_FACE('',(#1396),#1287,.T.);
#13965=ADVANCED_FACE('',(#1397),#13481,.T.);
#13966=ADVANCED_FACE('',(#1398),#1288,.F.);
#13967=ADVANCED_FACE('',(#1399,#641),#13482,.T.);
#13968=ADVANCED_FACE('',(#1400),#1289,.T.);
#13969=ADVANCED_FACE('',(#1401),#1290,.T.);
#13970=ADVANCED_FACE('',(#1402),#692,.T.);
#13971=ADVANCED_FACE('',(#1403),#693,.F.);
#13972=ADVANCED_FACE('',(#1404),#694,.F.);
#13973=ADVANCED_FACE('',(#1405),#13483,.T.);
#13974=ADVANCED_FACE('',(#1406),#695,.T.);
#13975=ADVANCED_FACE('',(#1407,#642),#13484,.T.);
#13976=ADVANCED_FACE('',(#1408),#13485,.T.);
#13977=ADVANCED_FACE('',(#1409,#643),#13486,.T.);
#14776=CLOSED_SHELL('',(#13936,#13937,#13938,#13939,#13940,#13941,#13942,
#13943,#13944,#13945,#13946,#13947,#13948,#13949,#13950,#13951,#13952,#13953,
#13954,#13955,#13956,#13957,#13958,#13959,#13960,#13961,#13962,#13963,#13964,
#13965,#13966,#13967,#13968,#13969,#13970,#13971,#13972,#13973,#13974,#13975,
#13976,#13977));
#14934=AXIS2_PLACEMENT_3D('',#19749,#16127,#16128);
#14935=AXIS2_PLACEMENT_3D('',#19750,#16129,#16130);
#14936=AXIS2_PLACEMENT_3D('',#19767,#16135,#16136);
#14937=AXIS2_PLACEMENT_3D('',#19777,#16140,#16141);
#14938=AXIS2_PLACEMENT_3D('',#19779,#16142,#16143);
#14939=AXIS2_PLACEMENT_3D('',#19788,#16144,#16145);
#14940=AXIS2_PLACEMENT_3D('',#19789,#16146,#16147);
#14941=AXIS2_PLACEMENT_3D('',#19791,#16148,#16149);
#14942=AXIS2_PLACEMENT_3D('',#19793,#16151,#16152);
#14943=AXIS2_PLACEMENT_3D('',#19797,#16155,#16156);
#14944=AXIS2_PLACEMENT_3D('',#19804,#16160,#16161);
#14945=AXIS2_PLACEMENT_3D('',#19810,#16165,#16166);
#14946=AXIS2_PLACEMENT_3D('',#19812,#16167,#16168);
#14947=AXIS2_PLACEMENT_3D('',#19815,#16170,#16171);
#14948=AXIS2_PLACEMENT_3D('',#19816,#16172,#16173);
#14949=AXIS2_PLACEMENT_3D('',#19824,#16176,#16177);
#14950=AXIS2_PLACEMENT_3D('',#19831,#16180,#16181);
#14951=AXIS2_PLACEMENT_3D('',#19834,#16184,#16185);
#14952=AXIS2_PLACEMENT_3D('',#19845,#16189,#16190);
#14953=AXIS2_PLACEMENT_3D('',#19847,#16191,#16192);
#14954=AXIS2_PLACEMENT_3D('',#19850,#16194,#16195);
#14955=AXIS2_PLACEMENT_3D('',#19851,#16196,#16197);
#14956=AXIS2_PLACEMENT_3D('',#19854,#16200,#16201);
#14957=AXIS2_PLACEMENT_3D('',#19856,#16202,#16203);
#14958=AXIS2_PLACEMENT_3D('',#19860,#16205,#16206);
#14959=AXIS2_PLACEMENT_3D('',#19865,#16209,#16210);
#14960=AXIS2_PLACEMENT_3D('',#19866,#16211,#16212);
#14961=AXIS2_PLACEMENT_3D('',#19868,#16214,#16215);
#14962=AXIS2_PLACEMENT_3D('',#19870,#16217,#16218);
#14963=AXIS2_PLACEMENT_3D('',#19881,#16220,#16221);
#14964=AXIS2_PLACEMENT_3D('',#19882,#16222,#16223);
#14965=AXIS2_PLACEMENT_3D('',#19892,#16227,#16228);
#14966=AXIS2_PLACEMENT_3D('',#19898,#16232,#16233);
#14967=AXIS2_PLACEMENT_3D('',#19902,#16236,#16237);
#14968=AXIS2_PLACEMENT_3D('',#19908,#16241,#16242);
#14969=AXIS2_PLACEMENT_3D('',#19913,#16244,#16245);
#14970=AXIS2_PLACEMENT_3D('',#19921,#16248,#16249);
#14971=AXIS2_PLACEMENT_3D('',#19923,#16250,#16251);
#14972=AXIS2_PLACEMENT_3D('',#19925,#16253,#16254);
#14973=AXIS2_PLACEMENT_3D('',#19927,#16256,#16257);
#14974=AXIS2_PLACEMENT_3D('',#19930,#16260,#16261);
#14975=AXIS2_PLACEMENT_3D('',#19936,#16265,#16266);
#14976=AXIS2_PLACEMENT_3D('',#19938,#16267,#16268);
#14977=AXIS2_PLACEMENT_3D('',#19941,#16270,#16271);
#14978=AXIS2_PLACEMENT_3D('',#19942,#16272,#16273);
#14979=AXIS2_PLACEMENT_3D('',#19950,#16276,#16277);
#14980=AXIS2_PLACEMENT_3D('',#19951,#16278,#16279);
#14981=AXIS2_PLACEMENT_3D('',#19953,#16280,#16281);
#14982=AXIS2_PLACEMENT_3D('',#19954,#16282,#16283);
#14983=AXIS2_PLACEMENT_3D('',#19959,#16284,#16285);
#14984=AXIS2_PLACEMENT_3D('',#19960,#16286,#16287);
#14985=AXIS2_PLACEMENT_3D('',#19965,#16288,#16289);
#14986=AXIS2_PLACEMENT_3D('',#19966,#16290,#16291);
#14987=AXIS2_PLACEMENT_3D('',#19967,#16292,#16293);
#14988=AXIS2_PLACEMENT_3D('',#19969,#16295,#16296);
#14989=AXIS2_PLACEMENT_3D('',#19972,#16298,#16299);
#14990=AXIS2_PLACEMENT_3D('',#19973,#16300,#16301);
#14991=AXIS2_PLACEMENT_3D('',#19975,#16302,#16303);
#14992=AXIS2_PLACEMENT_3D('',#19977,#16305,#16306);
#14993=AXIS2_PLACEMENT_3D('',#19978,#16307,#16308);
#14994=AXIS2_PLACEMENT_3D('',#19981,#16311,#16312);
#14995=AXIS2_PLACEMENT_3D('',#19982,#16313,#16314);
#14996=AXIS2_PLACEMENT_3D('',#19983,#16315,#16316);
#16127=DIRECTION('axis',(0.,0.,1.));
#16128=DIRECTION('refdir',(1.,0.,0.));
#16129=DIRECTION('center_axis',(-0.693904010166723,0.,-0.720067513969725));
#16130=DIRECTION('ref_axis',(-0.720067513969725,0.,0.693904010166723));
#16131=DIRECTION('',(0.591591578932266,-0.570096221587387,-0.570096221587386));
#16132=DIRECTION('',(0.,-1.,0.));
#16133=DIRECTION('',(-0.591591578932266,-0.570096221587387,0.570096221587386));
#16134=DIRECTION('',(0.,1.,0.));
#16135=DIRECTION('center_axis',(0.,0.707106781186547,-0.707106781186548));
#16136=DIRECTION('ref_axis',(-1.,0.,0.));
#16137=DIRECTION('',(1.,0.,0.));
#16138=DIRECTION('',(0.,-0.707106781186548,-0.707106781186547));
#16139=DIRECTION('',(-1.,0.,0.));
#16140=DIRECTION('center_axis',(0.,1.,0.));
#16141=DIRECTION('ref_axis',(1.,0.,0.));
#16142=DIRECTION('center_axis',(0.,-1.,0.));
#16143=DIRECTION('ref_axis',(1.,0.,0.));
#16144=DIRECTION('center_axis',(0.,1.,0.));
#16145=DIRECTION('ref_axis',(1.,0.,0.));
#16146=DIRECTION('center_axis',(0.,1.,0.));
#16147=DIRECTION('ref_axis',(1.,0.,0.));
#16148=DIRECTION('center_axis',(0.,1.,0.));
#16149=DIRECTION('ref_axis',(1.,0.,0.));
#16150=DIRECTION('',(0.,-1.,0.));
#16151=DIRECTION('center_axis',(0.577350269189625,0.577350269189626,-0.577350269189626));
#16152=DIRECTION('ref_axis',(-0.707106781186548,0.,-0.707106781186547));
#16153=DIRECTION('',(-0.707106781186547,0.707106781186547,4.08878244448899E-16));
#16154=DIRECTION('',(0.707106781186548,0.,0.707106781186547));
#16155=DIRECTION('center_axis',(0.577350269189625,-0.577350269189626,-0.577350269189626));
#16156=DIRECTION('ref_axis',(-0.707106781186548,0.,-0.707106781186547));
#16157=DIRECTION('',(-0.707106781186548,0.,-0.707106781186547));
#16158=DIRECTION('',(0.707106781186547,0.707106781186547,-4.08878244448899E-16));
#16159=DIRECTION('',(0.,-0.707106781186548,0.707106781186547));
#16160=DIRECTION('center_axis',(0.707106781186548,-0.707106781186548,0.));
#16161=DIRECTION('ref_axis',(0.,0.,-1.));
#16162=DIRECTION('',(-0.707106781186547,-0.707106781186547,0.));
#16163=DIRECTION('',(0.,0.,-1.));
#16164=DIRECTION('',(0.,0.,1.));
#16165=DIRECTION('center_axis',(0.,1.,0.));
#16166=DIRECTION('ref_axis',(0.707106781186549,0.,0.707106781186546));
#16167=DIRECTION('center_axis',(0.,-1.,0.));
#16168=DIRECTION('ref_axis',(0.707106781186549,0.,0.707106781186546));
#16169=DIRECTION('',(0.,-0.707106781186547,-0.707106781186548));
#16170=DIRECTION('center_axis',(0.,1.,0.));
#16171=DIRECTION('ref_axis',(0.707106781186549,0.,0.707106781186546));
#16172=DIRECTION('center_axis',(0.,-0.707106781186548,0.707106781186548));
#16173=DIRECTION('ref_axis',(1.,0.,0.));
#16174=DIRECTION('',(1.,0.,0.));
#16175=DIRECTION('',(-1.,0.,0.));
#16176=DIRECTION('center_axis',(0.,-0.707106781186547,-0.707106781186548));
#16177=DIRECTION('ref_axis',(-1.,0.,0.));
#16178=DIRECTION('',(1.,0.,0.));
#16179=DIRECTION('',(-1.,0.,0.));
#16180=DIRECTION('center_axis',(0.707106781186547,0.,-0.707106781186548));
#16181=DIRECTION('ref_axis',(-0.707106781186548,0.,-0.707106781186547));
#16182=DIRECTION('',(0.,-1.,0.));
#16183=DIRECTION('',(0.,1.,0.));
#16184=DIRECTION('center_axis',(0.,0.707106781186548,0.707106781186548));
#16185=DIRECTION('ref_axis',(1.,0.,0.));
#16186=DIRECTION('',(1.,0.,0.));
#16187=DIRECTION('',(0.,0.707106781186547,-0.707106781186547));
#16188=DIRECTION('',(-1.,0.,0.));
#16189=DIRECTION('center_axis',(0.,-1.,0.));
#16190=DIRECTION('ref_axis',(0.707106781186549,0.,0.707106781186546));
#16191=DIRECTION('center_axis',(0.,1.,0.));
#16192=DIRECTION('ref_axis',(0.707106781186549,0.,0.707106781186546));
#16193=DIRECTION('',(-0.707106781186547,0.707106781186547,-8.17756488897799E-16));
#16194=DIRECTION('center_axis',(0.,-1.,0.));
#16195=DIRECTION('ref_axis',(0.707106781186549,0.,0.707106781186546));
#16196=DIRECTION('center_axis',(0.707106781186548,0.707106781186548,0.));
#16197=DIRECTION('ref_axis',(0.,0.,-1.));
#16198=DIRECTION('',(0.,0.,-1.));
#16199=DIRECTION('',(0.,0.,1.));
#16200=DIRECTION('center_axis',(0.,1.,0.));
#16201=DIRECTION('ref_axis',(1.,0.,0.));
#16202=DIRECTION('center_axis',(0.,1.,0.));
#16203=DIRECTION('ref_axis',(1.,0.,0.));
#16204=DIRECTION('',(1.,0.,0.));
#16205=DIRECTION('center_axis',(0.,1.,0.));
#16206=DIRECTION('ref_axis',(-0.707106781186546,0.,0.707106781186549));
#16207=DIRECTION('',(0.,0.,1.));
#16208=DIRECTION('',(-1.,0.,0.));
#16209=DIRECTION('center_axis',(0.,-1.,0.));
#16210=DIRECTION('ref_axis',(1.,0.,0.));
#16211=DIRECTION('center_axis',(1.,0.,0.));
#16212=DIRECTION('ref_axis',(0.,0.,-1.));
#16213=DIRECTION('',(0.,1.,0.));
#16214=DIRECTION('center_axis',(0.,1.,0.));
#16215=DIRECTION('ref_axis',(0.707106781186549,0.,0.707106781186546));
#16216=DIRECTION('',(0.,-1.,0.));
#16217=DIRECTION('center_axis',(0.,0.,1.));
#16218=DIRECTION('ref_axis',(1.,0.,0.));
#16219=DIRECTION('',(0.,1.,0.));
#16220=DIRECTION('center_axis',(0.,0.,-1.));
#16221=DIRECTION('ref_axis',(1.,0.,0.));
#16222=DIRECTION('center_axis',(0.693904010166723,0.,-0.720067513969725));
#16223=DIRECTION('ref_axis',(-0.720067513969725,0.,-0.693904010166723));
#16224=DIRECTION('',(-0.591591578932266,0.570096221587387,-0.570096221587386));
#16225=DIRECTION('',(0.,1.,0.));
#16226=DIRECTION('',(0.591591578932266,0.570096221587387,0.570096221587386));
#16227=DIRECTION('center_axis',(0.,0.707106781186547,-0.707106781186548));
#16228=DIRECTION('ref_axis',(-1.,0.,0.));
#16229=DIRECTION('',(-1.,0.,0.));
#16230=DIRECTION('',(0.,0.707106781186548,0.707106781186547));
#16231=DIRECTION('',(1.,0.,0.));
#16232=DIRECTION('center_axis',(-0.577350269189626,0.577350269189626,-0.577350269189626));
#16233=DIRECTION('ref_axis',(-0.707106781186548,0.,0.707106781186547));
#16234=DIRECTION('',(0.707106781186548,0.,-0.707106781186547));
#16235=DIRECTION('',(-0.707106781186547,-0.707106781186547,4.08878244448899E-16));
#16236=DIRECTION('center_axis',(-0.577350269189626,-0.577350269189626,-0.577350269189626));
#16237=DIRECTION('ref_axis',(-0.707106781186548,0.,0.707106781186547));
#16238=DIRECTION('',(-0.707106781186548,0.,0.707106781186547));
#16239=DIRECTION('',(0.,0.707106781186548,-0.707106781186547));
#16240=DIRECTION('',(0.707106781186547,-0.707106781186547,-4.08878244448899E-16));
#16241=DIRECTION('center_axis',(0.,-0.707106781186547,-0.707106781186548));
#16242=DIRECTION('ref_axis',(-1.,0.,0.));
#16243=DIRECTION('',(1.,0.,0.));
#16244=DIRECTION('center_axis',(0.,-0.707106781186548,0.707106781186548));
#16245=DIRECTION('ref_axis',(1.,0.,0.));
#16246=DIRECTION('',(-1.,0.,0.));
#16247=DIRECTION('',(0.,-0.707106781186547,-0.707106781186547));
#16248=DIRECTION('center_axis',(0.,1.,0.));
#16249=DIRECTION('ref_axis',(-0.707106781186546,0.,0.707106781186549));
#16250=DIRECTION('center_axis',(0.,-1.,0.));
#16251=DIRECTION('ref_axis',(-0.707106781186546,0.,0.707106781186549));
#16252=DIRECTION('',(0.707106781186541,-0.707106781186554,0.));
#16253=DIRECTION('center_axis',(-0.707106781186548,-0.707106781186548,0.));
#16254=DIRECTION('ref_axis',(0.,0.,1.));
#16255=DIRECTION('',(0.,0.,-1.));
#16256=DIRECTION('center_axis',(-0.707106781186547,0.,-0.707106781186548));
#16257=DIRECTION('ref_axis',(-0.707106781186548,0.,0.707106781186547));
#16258=DIRECTION('',(0.,-1.,0.));
#16259=DIRECTION('',(0.,1.,0.));
#16260=DIRECTION('center_axis',(-0.707106781186548,0.707106781186548,0.));
#16261=DIRECTION('ref_axis',(0.,0.,1.));
#16262=DIRECTION('',(0.707106781186547,0.707106781186547,0.));
#16263=DIRECTION('',(0.,0.,-1.));
#16264=DIRECTION('',(0.,0.,1.));
#16265=DIRECTION('center_axis',(0.,-1.,0.));
#16266=DIRECTION('ref_axis',(-0.707106781186546,0.,0.707106781186549));
#16267=DIRECTION('center_axis',(0.,1.,0.));
#16268=DIRECTION('ref_axis',(-0.707106781186546,0.,0.707106781186549));
#16269=DIRECTION('',(0.,0.707106781186545,-0.70710678118655));
#16270=DIRECTION('center_axis',(0.,-1.,0.));
#16271=DIRECTION('ref_axis',(-0.707106781186546,0.,0.707106781186549));
#16272=DIRECTION('center_axis',(0.,0.707106781186548,0.707106781186548));
#16273=DIRECTION('ref_axis',(1.,0.,0.));
#16274=DIRECTION('',(-1.,0.,0.));
#16275=DIRECTION('',(1.,0.,0.));
#16276=DIRECTION('center_axis',(0.,-1.,0.));
#16277=DIRECTION('ref_axis',(1.,0.,0.));
#16278=DIRECTION('center_axis',(0.,0.,-1.));
#16279=DIRECTION('ref_axis',(-1.,0.,0.));
#16280=DIRECTION('center_axis',(0.,0.,1.));
#16281=DIRECTION('ref_axis',(1.,0.,0.));
#16282=DIRECTION('center_axis',(0.,1.,0.));
#16283=DIRECTION('ref_axis',(1.,0.,0.));
#16284=DIRECTION('center_axis',(0.,-1.,0.));
#16285=DIRECTION('ref_axis',(1.,0.,0.));
#16286=DIRECTION('center_axis',(0.,-1.,0.));
#16287=DIRECTION('ref_axis',(1.,0.,0.));
#16288=DIRECTION('center_axis',(0.,1.,0.));
#16289=DIRECTION('ref_axis',(1.,0.,0.));
#16290=DIRECTION('center_axis',(0.,-1.,0.));
#16291=DIRECTION('ref_axis',(1.,0.,0.));
#16292=DIRECTION('center_axis',(0.,1.,0.));
#16293=DIRECTION('ref_axis',(1.,0.,0.));
#16294=DIRECTION('',(0.,1.,0.));
#16295=DIRECTION('center_axis',(0.,0.,-1.));
#16296=DIRECTION('ref_axis',(1.,0.,0.));
#16297=DIRECTION('',(0.,0.,-1.));
#16298=DIRECTION('center_axis',(0.,0.,1.));
#16299=DIRECTION('ref_axis',(1.,0.,0.));
#16300=DIRECTION('center_axis',(0.,0.,-1.));
#16301=DIRECTION('ref_axis',(1.,0.,0.));
#16302=DIRECTION('center_axis',(0.,0.,-1.));
#16303=DIRECTION('ref_axis',(1.,0.,0.));
#16304=DIRECTION('',(0.,0.,-1.));
#16305=DIRECTION('center_axis',(0.,1.,0.));
#16306=DIRECTION('ref_axis',(1.,0.,0.));
#16307=DIRECTION('center_axis',(0.,1.,0.));
#16308=DIRECTION('ref_axis',(-0.707106781186546,0.,0.707106781186549));
#16309=DIRECTION('',(0.,1.,0.));
#16310=DIRECTION('',(0.,-1.,0.));
#16311=DIRECTION('center_axis',(0.,0.,1.));
#16312=DIRECTION('ref_axis',(1.,0.,0.));
#16313=DIRECTION('center_axis',(-1.,0.,0.));
#16314=DIRECTION('ref_axis',(0.,0.,1.));
#16315=DIRECTION('center_axis',(0.,0.,-1.));
#16316=DIRECTION('ref_axis',(-1.,0.,0.));
#19749=CARTESIAN_POINT('',(0.,0.,0.));
#19750=CARTESIAN_POINT('Origin',(20.2248703552884,-6.,0.7398357130565));
#19751=CARTESIAN_POINT('',(20.2359894539709,5.74912062451897,0.729120624518965));
#19752=CARTESIAN_POINT('',(20.4737490231322,5.52,0.5));
#19753=CARTESIAN_POINT('',(16.044254314835,9.78854993659521,4.7685499365952));
#19754=CARTESIAN_POINT('',(20.4737490231322,-5.52,0.5));
#19755=CARTESIAN_POINT('',(20.4737490231322,-6.,0.5));
#19756=CARTESIAN_POINT('',(20.2359894539709,-5.74912062451896,0.72912062451896));
#19757=CARTESIAN_POINT('',(14.0206695716018,-11.7386081478045,6.71860814780449));
#19758=CARTESIAN_POINT('',(19.9759916874447,-5.5,0.979671426113));
#19759=CARTESIAN_POINT('Ctrl Pts',(20.2359894539709,-5.74912062451896,0.72912062451896));
#19760=CARTESIAN_POINT('Ctrl Pts',(20.1051859468429,-5.62294071733703,0.855171413339531));
#19761=CARTESIAN_POINT('Ctrl Pts',(19.9759916874447,-5.5,0.979671426112999));
#19762=CARTESIAN_POINT('',(19.9759916874447,5.5,0.979671426113));
#19763=CARTESIAN_POINT('',(19.9759916874447,-6.,0.979671426113));
#19764=CARTESIAN_POINT('Ctrl Pts',(19.9759916874446,5.5,0.979671426113002));
#19765=CARTESIAN_POINT('Ctrl Pts',(20.1051859468428,5.6229407173369,0.855171413339668));
#19766=CARTESIAN_POINT('Ctrl Pts',(20.2359894539709,5.74912062451897,0.729120624518965));
#19767=CARTESIAN_POINT('Origin',(-14.9979165219706,5.76,0.74));
#19768=CARTESIAN_POINT('',(20.4765622114651,6.,0.98));
#19769=CARTESIAN_POINT('Ctrl Pts',(20.2359894539709,5.74912062451897,0.729120624518965));
#19770=CARTESIAN_POINT('Ctrl Pts',(20.3562758327179,5.87381908208973,0.853819082089724));
#19771=CARTESIAN_POINT('Ctrl Pts',(20.4765622114651,6.,0.98));
#19772=CARTESIAN_POINT('',(45.17,6.,0.98));
#19773=CARTESIAN_POINT('',(-14.9979165219706,6.,0.98));
#19774=CARTESIAN_POINT('',(45.17,5.52,0.5));
#19775=CARTESIAN_POINT('',(45.17,6.,0.98));
#19776=CARTESIAN_POINT('',(-14.9979165219706,5.52,0.5));
#19777=CARTESIAN_POINT('Origin',(0.,5.75,0.));
#19778=CARTESIAN_POINT('',(-19.9759916874447,5.5,0.979671426113));
#19779=CARTESIAN_POINT('Origin',(0.,5.5,0.));
#19780=CARTESIAN_POINT('',(-20.2359894539709,5.74912062451897,0.729120624518964));
#19781=CARTESIAN_POINT('Ctrl Pts',(-20.2359894539709,5.74912062451897,0.729120624518964));
#19782=CARTESIAN_POINT('Ctrl Pts',(-20.105185946843,5.62294071733708,0.855171413339494));
#19783=CARTESIAN_POINT('Ctrl Pts',(-19.9759916874447,5.5,0.979671426113));
#19784=CARTESIAN_POINT('',(-20.4765622114651,6.,0.98));
#19785=CARTESIAN_POINT('Ctrl Pts',(-20.4765622114651,6.,0.98));
#19786=CARTESIAN_POINT('Ctrl Pts',(-20.356275832718,5.87381908208979,0.853819082089789));
#19787=CARTESIAN_POINT('Ctrl Pts',(-20.2359894539709,5.74912062451897,0.729120624518963));
#19788=CARTESIAN_POINT('Origin',(0.,6.,0.));
#19789=CARTESIAN_POINT('Origin',(0.,-6.,0.));
#19790=CARTESIAN_POINT('',(-19.9759916874447,-5.5,0.979671426113));
#19791=CARTESIAN_POINT('Origin',(0.,-5.5,0.));
#19792=CARTESIAN_POINT('',(-19.9759916874447,-6.,0.979671426113));
#19793=CARTESIAN_POINT('Origin',(45.17,5.52,0.5));
#19794=CARTESIAN_POINT('',(45.65,5.52,0.98));
#19795=CARTESIAN_POINT('',(45.65,5.52,0.98));
#19796=CARTESIAN_POINT('',(45.17,5.52,0.5));
#19797=CARTESIAN_POINT('Origin',(45.17,-6.,0.98));
#19798=CARTESIAN_POINT('',(45.65,-5.52,0.98));
#19799=CARTESIAN_POINT('',(45.17,-5.52,0.5));
#19800=CARTESIAN_POINT('',(45.65,-5.52,0.98));
#19801=CARTESIAN_POINT('',(45.17,-6.,0.98));
#19802=CARTESIAN_POINT('',(45.17,-6.,0.98));
#19803=CARTESIAN_POINT('',(45.17,-5.52,0.5));
#19804=CARTESIAN_POINT('Origin',(45.41,-5.76,3.));
#19805=CARTESIAN_POINT('',(45.65,-5.52,4.));
#19806=CARTESIAN_POINT('',(45.17,-6.,4.));
#19807=CARTESIAN_POINT('',(45.65,-5.52,4.));
#19808=CARTESIAN_POINT('',(45.17,-6.,3.));
#19809=CARTESIAN_POINT('',(45.65,-5.52,3.));
#19810=CARTESIAN_POINT('Origin',(43.65,-5.76,4.));
#19811=CARTESIAN_POINT('',(43.65,-5.52,6.));
#19812=CARTESIAN_POINT('Origin',(43.65,-5.52,4.));
#19813=CARTESIAN_POINT('',(43.65,-6.,5.52));
#19814=CARTESIAN_POINT('',(43.65,-5.52,6.));
#19815=CARTESIAN_POINT('Origin',(43.65,-6.,4.));
#19816=CARTESIAN_POINT('Origin',(14.6969384566991,-5.76,5.76));
#19817=CARTESIAN_POINT('',(29.3734642151722,-5.52,6.));
#19818=CARTESIAN_POINT('',(28.9789509817039,-6.,5.52));
#19819=CARTESIAN_POINT('Ctrl Pts',(28.9789509817039,-6.,5.52));
#19820=CARTESIAN_POINT('Ctrl Pts',(29.1762075984394,-5.76162260937474,5.75837739062526));
#19821=CARTESIAN_POINT('Ctrl Pts',(29.3734642151722,-5.52,6.));
#19822=CARTESIAN_POINT('',(14.6969384566991,-6.,5.52));
#19823=CARTESIAN_POINT('',(14.6969384566991,-5.52,6.));
#19824=CARTESIAN_POINT('Origin',(-14.9979165219706,-5.76,0.74));
#19825=CARTESIAN_POINT('',(-14.9979165219706,-5.52,0.5));
#19826=CARTESIAN_POINT('',(20.4765622114651,-6.,0.98));
#19827=CARTESIAN_POINT('',(-14.9979165219706,-6.,0.98));
#19828=CARTESIAN_POINT('Ctrl Pts',(20.4765622114651,-6.,0.98));
#19829=CARTESIAN_POINT('Ctrl Pts',(20.356275832718,-5.87381908208979,0.853819082089787));
#19830=CARTESIAN_POINT('Ctrl Pts',(20.2359894539709,-5.74912062451896,0.729120624518961));
#19831=CARTESIAN_POINT('Origin',(45.41,-6.,0.74));
#19832=CARTESIAN_POINT('',(45.65,-6.,0.98));
#19833=CARTESIAN_POINT('',(45.17,-6.,0.5));
#19834=CARTESIAN_POINT('Origin',(14.6969384566991,5.76,5.76));
#19835=CARTESIAN_POINT('',(28.9789509817039,6.,5.52));
#19836=CARTESIAN_POINT('',(29.3734642151722,5.52,6.));
#19837=CARTESIAN_POINT('Ctrl Pts',(29.3734642151722,5.52,6.));
#19838=CARTESIAN_POINT('Ctrl Pts',(29.1762075984394,5.76162260937474,5.75837739062526));
#19839=CARTESIAN_POINT('Ctrl Pts',(28.9789509817039,6.,5.52));
#19840=CARTESIAN_POINT('',(43.65,5.52,6.));
#19841=CARTESIAN_POINT('',(14.6969384566991,5.52,6.));
#19842=CARTESIAN_POINT('',(43.65,6.,5.52));
#19843=CARTESIAN_POINT('',(43.65,5.52,6.));
#19844=CARTESIAN_POINT('',(14.6969384566991,6.,5.52));
#19845=CARTESIAN_POINT('Origin',(43.65,5.76,4.));
#19846=CARTESIAN_POINT('',(45.65,5.52,4.));
#19847=CARTESIAN_POINT('Origin',(43.65,5.52,4.));
#19848=CARTESIAN_POINT('',(45.17,6.,4.));
#19849=CARTESIAN_POINT('',(45.65,5.52,4.));
#19850=CARTESIAN_POINT('Origin',(43.65,6.,4.));
#19851=CARTESIAN_POINT('Origin',(45.41,5.76,3.));
#19852=CARTESIAN_POINT('',(45.65,5.52,3.));
#19853=CARTESIAN_POINT('',(45.17,6.,3.));
#19854=CARTESIAN_POINT('Origin',(0.,-6.,0.));
#19855=CARTESIAN_POINT('',(-28.9789509817039,-6.,5.52));
#19856=CARTESIAN_POINT('Origin',(0.,-6.,0.));
#19857=CARTESIAN_POINT('',(-43.65,-6.,5.52));
#19858=CARTESIAN_POINT('',(-22.825,-6.,5.52));
#19859=CARTESIAN_POINT('',(-45.17,-6.,4.));
#19860=CARTESIAN_POINT('Origin',(-43.65,-6.,4.));
#19861=CARTESIAN_POINT('',(-45.17,-6.,0.98));
#19862=CARTESIAN_POINT('',(-45.17,-6.,0.25));
#19863=CARTESIAN_POINT('',(-20.4765622114651,-6.,0.98));
#19864=CARTESIAN_POINT('',(-14.9979165219706,-6.,0.98));
#19865=CARTESIAN_POINT('Origin',(0.,-6.,0.));
#19866=CARTESIAN_POINT('Origin',(45.65,-6.,6.));
#19867=CARTESIAN_POINT('',(45.65,-6.,4.));
#19868=CARTESIAN_POINT('Origin',(43.65,-6.,4.));
#19869=CARTESIAN_POINT('',(43.65,-6.,6.));
#19870=CARTESIAN_POINT('Origin',(29.3938769133981,-6.,6.));
#19871=CARTESIAN_POINT('',(29.3938769133981,5.5,6.));
#19872=CARTESIAN_POINT('Ctrl Pts',(29.3734642151722,5.51999999999998,6.));
#19873=CARTESIAN_POINT('Ctrl Pts',(29.3836671610351,5.51000347347589,6.));
#19874=CARTESIAN_POINT('Ctrl Pts',(29.3938769133981,5.5,6.));
#19875=CARTESIAN_POINT('',(29.3938769133981,-5.5,6.));
#19876=CARTESIAN_POINT('',(29.3938769133981,-6.,6.));
#19877=CARTESIAN_POINT('Ctrl Pts',(29.3938769133981,-5.5,6.));
#19878=CARTESIAN_POINT('Ctrl Pts',(29.3836671610351,-5.51000347347589,6.));
#19879=CARTESIAN_POINT('Ctrl Pts',(29.3734642151722,-5.51999999999997,6.));
#19880=CARTESIAN_POINT('',(37.25,-2.75545529808154E-16,6.));
#19881=CARTESIAN_POINT('Origin',(39.5,0.,6.));
#19882=CARTESIAN_POINT('Origin',(-20.2248703552884,-6.,0.7398357130565));
#19883=CARTESIAN_POINT('',(-20.2359894539709,-5.74912062451896,0.729120624518962));
#19884=CARTESIAN_POINT('',(-20.4737490231322,-5.52,0.5));
#19885=CARTESIAN_POINT('',(-19.2696493386723,-6.68034897211366,1.66034897211366));
#19886=CARTESIAN_POINT('',(-20.4737490231322,5.52,0.5));
#19887=CARTESIAN_POINT('',(-20.4737490231322,-6.,0.5));
#19888=CARTESIAN_POINT('',(-21.2932340819055,4.73029076090437,-0.289709239095627));
#19889=CARTESIAN_POINT('Ctrl Pts',(-19.9759916874447,-5.5,0.979671426112999));
#19890=CARTESIAN_POINT('Ctrl Pts',(-20.1051859468429,-5.62294071733703,
0.855171413339532));
#19891=CARTESIAN_POINT('Ctrl Pts',(-20.2359894539709,-5.74912062451896,
0.729120624518962));
#19892=CARTESIAN_POINT('Origin',(-14.9979165219706,5.76,0.74));
#19893=CARTESIAN_POINT('',(-45.17,5.52,0.5));
#19894=CARTESIAN_POINT('',(-14.9979165219706,5.52,0.5));
#19895=CARTESIAN_POINT('',(-45.17,6.,0.98));
#19896=CARTESIAN_POINT('',(-45.17,5.52,0.5));
#19897=CARTESIAN_POINT('',(-14.9979165219706,6.,0.98));
#19898=CARTESIAN_POINT('Origin',(-45.65,5.52,0.98));
#19899=CARTESIAN_POINT('',(-45.65,5.52,0.98));
#19900=CARTESIAN_POINT('',(-45.65,5.52,0.98));
#19901=CARTESIAN_POINT('',(-45.17,6.,0.98));
#19902=CARTESIAN_POINT('Origin',(-45.17,-6.,0.98));
#19903=CARTESIAN_POINT('',(-45.17,-5.52,0.5));
#19904=CARTESIAN_POINT('',(-45.65,-5.52,0.98));
#19905=CARTESIAN_POINT('',(-45.17,-5.52,0.5));
#19906=CARTESIAN_POINT('',(-45.17,-6.,0.98));
#19907=CARTESIAN_POINT('',(-45.65,-5.52,0.98));
#19908=CARTESIAN_POINT('Origin',(-14.9979165219706,-5.76,0.74));
#19909=CARTESIAN_POINT('Ctrl Pts',(-20.2359894539709,-5.74912062451896,
0.729120624518962));
#19910=CARTESIAN_POINT('Ctrl Pts',(-20.3562758327179,-5.87381908208974,
0.853819082089735));
#19911=CARTESIAN_POINT('Ctrl Pts',(-20.4765622114651,-6.,0.98));
#19912=CARTESIAN_POINT('',(-14.9979165219706,-5.52,0.5));
#19913=CARTESIAN_POINT('Origin',(-22.825,-5.76,5.76));
#19914=CARTESIAN_POINT('',(-29.3734642151722,-5.52,6.));
#19915=CARTESIAN_POINT('Ctrl Pts',(-29.3734642151722,-5.52,6.));
#19916=CARTESIAN_POINT('Ctrl Pts',(-29.1762075984394,-5.76162260937474,
5.75837739062526));
#19917=CARTESIAN_POINT('Ctrl Pts',(-28.9789509817039,-6.,5.52));
#19918=CARTESIAN_POINT('',(-43.65,-5.52,6.));
#19919=CARTESIAN_POINT('',(-22.825,-5.52,6.));
#19920=CARTESIAN_POINT('',(-43.65,-5.52,6.));
#19921=CARTESIAN_POINT('Origin',(-43.65,-5.76,4.));
#19922=CARTESIAN_POINT('',(-45.65,-5.52,4.));
#19923=CARTESIAN_POINT('Origin',(-43.65,-5.52,4.));
#19924=CARTESIAN_POINT('',(-45.65,-5.52,4.));
#19925=CARTESIAN_POINT('Origin',(-45.41,-5.76,0.25));
#19926=CARTESIAN_POINT('',(-45.65,-5.52,0.25));
#19927=CARTESIAN_POINT('Origin',(-45.41,-6.,0.74));
#19928=CARTESIAN_POINT('',(-45.17,-6.,0.5));
#19929=CARTESIAN_POINT('',(-45.65,-6.,0.98));
#19930=CARTESIAN_POINT('Origin',(-45.41,5.76,0.25));
#19931=CARTESIAN_POINT('',(-45.65,5.52,4.));
#19932=CARTESIAN_POINT('',(-45.17,6.,4.));
#19933=CARTESIAN_POINT('',(-45.65,5.52,4.));
#19934=CARTESIAN_POINT('',(-45.17,6.,0.25));
#19935=CARTESIAN_POINT('',(-45.65,5.52,0.25));
#19936=CARTESIAN_POINT('Origin',(-43.65,5.76,4.));
#19937=CARTESIAN_POINT('',(-43.65,5.52,6.));
#19938=CARTESIAN_POINT('Origin',(-43.65,5.52,4.));
#19939=CARTESIAN_POINT('',(-43.65,6.,5.52));
#19940=CARTESIAN_POINT('',(-43.65,5.52,6.));
#19941=CARTESIAN_POINT('Origin',(-43.65,6.,4.));
#19942=CARTESIAN_POINT('Origin',(-22.825,5.76,5.76));
#19943=CARTESIAN_POINT('',(-29.3734642151722,5.52,6.));
#19944=CARTESIAN_POINT('',(-28.9789509817039,6.,5.52));
#19945=CARTESIAN_POINT('Ctrl Pts',(-28.9789509817039,6.,5.52));
#19946=CARTESIAN_POINT('Ctrl Pts',(-29.1762075984394,5.76162260937474,5.75837739062526));
#19947=CARTESIAN_POINT('Ctrl Pts',(-29.3734642151722,5.52,6.));
#19948=CARTESIAN_POINT('',(-22.825,6.,5.52));
#19949=CARTESIAN_POINT('',(-22.825,5.52,6.));
#19950=CARTESIAN_POINT('Origin',(0.,-5.75,0.));
#19951=CARTESIAN_POINT('Origin',(-29.9958330439413,-6.,0.5));
#19952=CARTESIAN_POINT('',(-41.75,-2.75545529808155E-16,0.5));
#19953=CARTESIAN_POINT('Origin',(-39.5,0.,0.5));
#19954=CARTESIAN_POINT('Origin',(0.,-5.75,0.));
#19955=CARTESIAN_POINT('',(-29.3938769133981,-5.5,6.));
#19956=CARTESIAN_POINT('Ctrl Pts',(-29.3734642151722,-5.51999999999998,
6.));
#19957=CARTESIAN_POINT('Ctrl Pts',(-29.3836671610351,-5.51000347347589,
6.));
#19958=CARTESIAN_POINT('Ctrl Pts',(-29.3938769133981,-5.5,6.));
#19959=CARTESIAN_POINT('Origin',(0.,-5.5,0.));
#19960=CARTESIAN_POINT('Origin',(0.,5.75,0.));
#19961=CARTESIAN_POINT('',(-29.3938769133981,5.5,6.));
#19962=CARTESIAN_POINT('Ctrl Pts',(-29.3938769133981,5.5,6.));
#19963=CARTESIAN_POINT('Ctrl Pts',(-29.3836671610351,5.51000347347589,6.));
#19964=CARTESIAN_POINT('Ctrl Pts',(-29.3734642151722,5.51999999999998,6.));
#19965=CARTESIAN_POINT('Origin',(0.,5.5,0.));
#19966=CARTESIAN_POINT('Origin',(0.,6.,0.));
#19967=CARTESIAN_POINT('Origin',(0.,-6.,0.));
#19968=CARTESIAN_POINT('',(-29.3938769133981,-6.,6.));
#19969=CARTESIAN_POINT('Origin',(39.5,0.,6.));
#19970=CARTESIAN_POINT('',(37.25,-2.75545529808154E-16,0.5));
#19971=CARTESIAN_POINT('',(37.25,2.75545529808154E-16,6.));
#19972=CARTESIAN_POINT('Origin',(39.5,0.,0.5));
#19973=CARTESIAN_POINT('Origin',(-39.5,0.,6.));
#19974=CARTESIAN_POINT('',(-41.75,-2.75545529808155E-16,6.));
#19975=CARTESIAN_POINT('Origin',(-39.5,0.,6.));
#19976=CARTESIAN_POINT('',(-41.75,2.75545529808155E-16,6.));
#19977=CARTESIAN_POINT('Origin',(0.,6.,0.));
#19978=CARTESIAN_POINT('Origin',(-43.65,-6.,4.));
#19979=CARTESIAN_POINT('',(-43.65,-6.,6.));
#19980=CARTESIAN_POINT('',(-45.65,-6.,4.));
#19981=CARTESIAN_POINT('Origin',(-45.65,-6.,6.));
#19982=CARTESIAN_POINT('Origin',(-45.65,-6.,0.5));
#19983=CARTESIAN_POINT('Origin',(-29.9958330439413,-6.,0.5));
#37153=UNCERTAINTY_MEASURE_WITH_UNIT(LENGTH_MEASURE(0.01),#37182,
'DISTANCE_ACCURACY_VALUE',
'Maximum model space distance between geometric entities at asserted c
onnectivities');
#37166=UNCERTAINTY_MEASURE_WITH_UNIT(LENGTH_MEASURE(0.01),#37182,
'DISTANCE_ACCURACY_VALUE',
'Maximum model space distance between geometric entities at asserted c
onnectivities');
#37168=(
GEOMETRIC_REPRESENTATION_CONTEXT(3)
GLOBAL_UNCERTAINTY_ASSIGNED_CONTEXT((#37153))
GLOBAL_UNIT_ASSIGNED_CONTEXT((#37182,#37184,#37185))
REPRESENTATION_CONTEXT('','3D')
);
#37181=(
GEOMETRIC_REPRESENTATION_CONTEXT(3)
GLOBAL_UNCERTAINTY_ASSIGNED_CONTEXT((#37166))
GLOBAL_UNIT_ASSIGNED_CONTEXT((#37182,#37184,#37185))
REPRESENTATION_CONTEXT('','3D')
);
#37182=(
LENGTH_UNIT()
NAMED_UNIT(*)
SI_UNIT(.MILLI.,.METRE.)
);
#37184=(
NAMED_UNIT(*)
PLANE_ANGLE_UNIT()
SI_UNIT($,.RADIAN.)
);
#37185=(
NAMED_UNIT(*)
SI_UNIT($,.STERADIAN.)
SOLID_ANGLE_UNIT()
);
#37187=SHAPE_DEFINITION_REPRESENTATION(#37201,#37238);
#37201=PRODUCT_DEFINITION_SHAPE('',$,#37253);
#37238=SHAPE_REPRESENTATION('',(#14934),#37168);
#37251=PRODUCT_DEFINITION_CONTEXT('part definition',#37295,'design');
#37253=PRODUCT_DEFINITION('2026-10-20-13-23-47-382',
'01_Clamp_Upper_Half_PLA',#37267,#37251);
#37267=PRODUCT_DEFINITION_FORMATION('',$,#37298);
#37295=APPLICATION_CONTEXT(
'Core Data for Automotive Mechanical Design Process');
#37296=PRODUCT_CONTEXT('part definition',#37295,'mechanical');
#37298=PRODUCT('2026-10-20-13-23-47-382','01_Clamp_Upper_Half_PLA',$,(#37296));
#37353=COLOUR_RGB('Light Blue',0.38,0.62,0.78);
#37354=FILL_AREA_STYLE_COLOUR('',#37353);
#37355=FILL_AREA_STYLE('',(#37354));
#37356=SURFACE_STYLE_FILL_AREA(#37355);
#37357=SURFACE_SIDE_STYLE('',(#37356));
#37358=SURFACE_STYLE_USAGE(.BOTH.,#37357);
#37359=PRESENTATION_STYLE_ASSIGNMENT((#37358));
ENDSEC;
END-ISO-10303-21;
